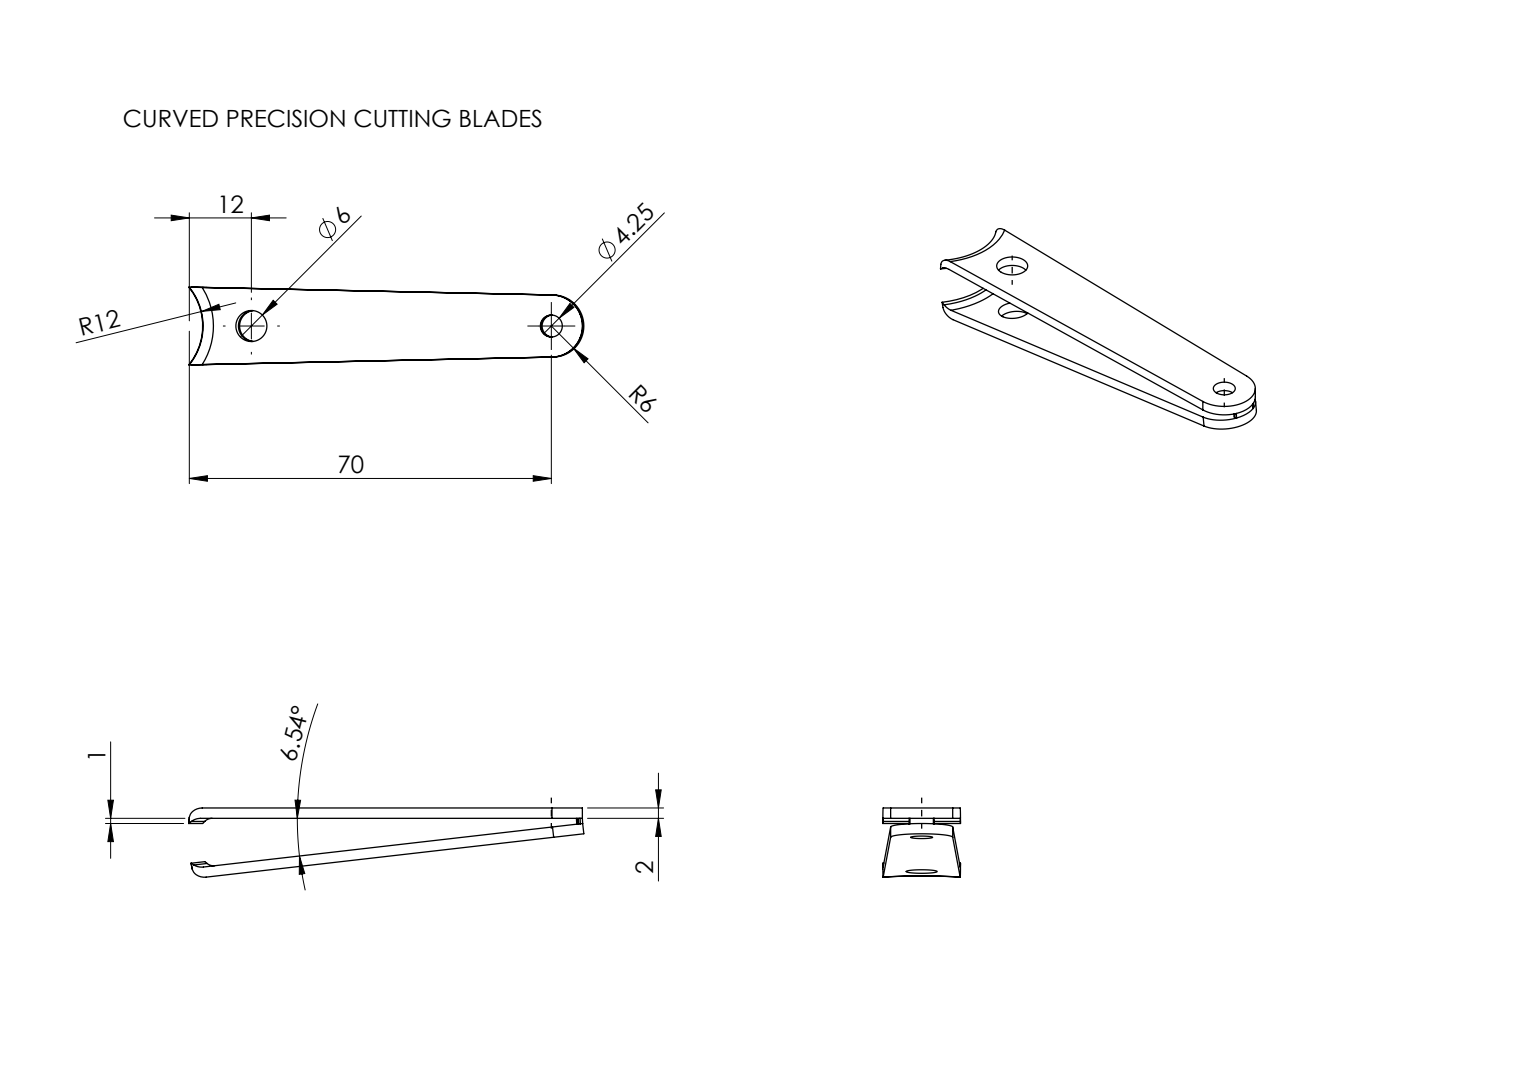
ISO-10303-21;
HEADER;
FILE_DESCRIPTION (('STEP AP214'),
    '1' );
FILE_NAME ('Curved Precision Cutting Blades.step',
    '2026-09-30T04:43:20',
    ( '' ),
    ( '' ),
    'SwSTEP 2.0',
    'SolidWorks 2026',
    '' );
FILE_SCHEMA (( 'AUTOMOTIVE_DESIGN' ));
ENDSEC;

DATA;
#18=VERTEX_POINT ( 'NONE', #46192 ) ;
#27=B_SPLINE_CURVE_WITH_KNOTS ( 'NONE', 3,
 ( #5781, #31047, #23391, #22809, #48941, #35902, #48672, #40707, #18006, #52911, #26803, #36426 ),
 .UNSPECIFIED., .F., .F.,
 ( 4, 2, 2, 2, 2, 4 ),
 ( 0.07980989636644560126, 0.1159099261691615840, 0.2318198523383231402, 0.4636397046766463914, 0.6954595570149695316, 0.9272794093314227215 ),
 .UNSPECIFIED. ) ;
#61=CARTESIAN_POINT ( 'NONE',  ( -69.74692240850775704, 2.000000000000830003, -7.382776467523781250 ) ) ;
#63=ORIENTED_EDGE ( 'NONE', *, *, #47329, .F. ) ;
#89=EDGE_CURVE ( 'NONE', #51823, #2618, #23778, .T. ) ;
#128=ORIENTED_EDGE ( 'NONE', *, *, #52773, .T. ) ;
#145=AXIS2_PLACEMENT_3D ( 'NONE', #38403, #43503, #3755 ) ;
#186=CARTESIAN_POINT ( 'NONE',  ( -66.51694242614880181, -11.33548347488676278, 2.024546322512585039 ) ) ;
#253=ORIENTED_EDGE ( 'NONE', *, *, #19870, .F. ) ;
#280=VERTEX_POINT ( 'NONE', #756 ) ;
#299=DIRECTION ( 'NONE',  ( -0.1139275668495183524, 0.9934890585767659488, 4.694855797473114533E-16 ) ) ;
#354=CARTESIAN_POINT ( 'NONE',  ( -69.95337746243399124, 0.1332479302464926740, -7.442420802399271729 ) ) ;
#433=CARTESIAN_POINT ( 'NONE',  ( 0.4518049228021103203, -3.655895688227122076, 5.998622290806040702 ) ) ;
#492=DIRECTION ( 'NONE',  ( -0.9997703818010067467, 0.000000000000000000, -0.02142857142857158143 ) ) ;
#495=CARTESIAN_POINT ( 'NONE',  ( 4.866417447938704122, 0.000000000000000000, 1.967953638241001002 ) ) ;
#496=CARTESIAN_POINT ( 'NONE',  ( 6.057149706651311583, -1.000000014492634426, -0.7725429650402538817 ) ) ;
#563=VERTEX_POINT ( 'NONE', #20602 ) ;
#641=CARTESIAN_POINT ( 'NONE',  ( -69.63135658628988267, 1.044799017367015193, 7.493821216008851316 ) ) ;
#653=CARTESIAN_POINT ( 'NONE',  ( 4.930947970565944694, -1.129146301979397693, 1.967953638241001446 ) ) ;
#674=ORIENTED_EDGE ( 'NONE', *, *, #1413, .T. ) ;
#685=( BOUNDED_SURFACE ( )  B_SPLINE_SURFACE ( 3, 2, ( 
 ( #15116, #40673, #41213 ),
 ( #40925, #15367, #2009 ),
 ( #44927, #36680, #10586 ),
 ( #28148, #36390, #6041 ),
 ( #45740, #50283, #49989 ),
 ( #19904, #11101, #45457 ),
 ( #10837, #28728, #2308 ),
 ( #24185, #6868, #23354 ),
 ( #1745, #11397, #28423 ),
 ( #45205, #10278, #53441 ),
 ( #19067, #14539, #27899 ),
 ( #6572, #36975, #5739 ),
 ( #23063, #6307, #41503 ),
 ( #54273, #19644, #32439 ),
 ( #32683, #2586, #37220 ),
 ( #53703, #54524, #40385 ),
 ( #49165, #15631, #14818 ),
 ( #32970, #27603, #31853 ),
 ( #1480, #32145, #49470 ),
 ( #18819, #23610, #19344 ),
 ( #53999, #36140, #49740 ),
 ( #23885, #12789, #11933 ),
 ( #42345, #38343, #25300 ),
 ( #33807, #42604, #51427 ),
 ( #41750, #37811, #12527 ),
 ( #7144, #33274, #34109 ),
 ( #3698, #29846, #24716 ),
 ( #54824, #34380, #55668 ) ),
 .UNSPECIFIED., .F., .F., .T. ) 
 B_SPLINE_SURFACE_WITH_KNOTS ( ( 4, 2, 2, 2, 2, 2, 2, 2, 2, 2, 2, 2, 2, 4 ),
 ( 3, 3 ),
 ( 0.005951394764495079696, 0.008223488340404871977, 0.009359535128359769418, 0.01049558191631466512, 0.01276767549222445827, 0.01390372228017935571, 0.01503976906813425142, 0.01617581585608914713, 0.01731186264404404457, 0.01958395621995383598, 0.02072000300790872995, 0.02185604979586362739, 0.02299209658381852484, 0.02412814337177342228 ),
 ( 0.000000000000000000, 1.000000000000000000 ),
 .UNSPECIFIED. ) 
 GEOMETRIC_REPRESENTATION_ITEM ( )  RATIONAL_B_SPLINE_SURFACE ( (
 ( 1.000000000000000000, 0.9218171296615420562, 1.000000000000000000),
 ( 1.000000000000000000, 0.9219582590456437687, 1.000000000000000000),
 ( 1.000000000000000000, 0.9217654209472763149, 1.000000000000000000),
 ( 1.000000000000000000, 0.9218193965238216103, 1.000000000000000000),
 ( 1.000000000000000000, 0.9217886515250015567, 1.000000000000000000),
 ( 1.000000000000000000, 0.9217705453232085677, 1.000000000000000000),
 ( 1.000000000000000000, 0.9217728555239398380, 1.000000000000000000),
 ( 1.000000000000000000, 0.9217839018313299659, 1.000000000000000000),
 ( 1.000000000000000000, 0.9217902773711394993, 1.000000000000000000),
 ( 1.000000000000000000, 0.9218159477363486731, 1.000000000000000000),
 ( 1.000000000000000000, 0.9218381644591753243, 1.000000000000000000),
 ( 1.000000000000000000, 0.9218170478689924341, 1.000000000000000000),
 ( 1.000000000000000000, 0.9218183721981643153, 1.000000000000000000),
 ( 1.000000000000000000, 0.9218243750428467553, 1.000000000000000000),
 ( 1.000000000000000000, 0.9218291361982778875, 1.000000000000000000),
 ( 1.000000000000000000, 0.9218339850783857647, 1.000000000000000000),
 ( 1.000000000000000000, 0.9218340914611712344, 1.000000000000000000),
 ( 1.000000000000000000, 0.9218311426327383540, 1.000000000000000000),
 ( 1.000000000000000000, 0.9218408506515718415, 1.000000000000000000),
 ( 1.000000000000000000, 0.9218298856236216698, 1.000000000000000000),
 ( 1.000000000000000000, 0.9218235216668148047, 1.000000000000000000),
 ( 1.000000000000000000, 0.9218049054835019129, 1.000000000000000000),
 ( 1.000000000000000000, 0.9217926302239767278, 1.000000000000000000),
 ( 1.000000000000000000, 0.9217749384505029564, 1.000000000000000000),
 ( 1.000000000000000000, 0.9217695517188592147, 1.000000000000000000),
 ( 1.000000000000000000, 0.9217886187906866313, 1.000000000000000000),
 ( 1.000000000000000000, 0.9218984684751942993, 1.000000000000000000),
 ( 1.000000000000000000, 0.9217608302862917435, 1.000000000000000000) ) ) 
 REPRESENTATION_ITEM ( '' )  SURFACE ( )  );
#689=CYLINDRICAL_SURFACE ( 'NONE', #24963, 5.241923709989091407 ) ;
#709=CARTESIAN_POINT ( 'NONE',  ( -70.02519189693502710, -0.1222117011752772570, -7.502262482362483276 ) ) ;
#756=CARTESIAN_POINT ( 'NONE',  ( -57.52614991588065152, -8.291364278369169227, 3.000000000000006661 ) ) ;
#761=CARTESIAN_POINT ( 'NONE',  ( -67.73103538350329700, -11.31014138737506336, -7.469194291234003913 ) ) ;
#771=CARTESIAN_POINT ( 'NONE',  ( 6.057149959413268725, -0.9999999855073579136, 0.7725409890818936143 ) ) ;
#933=ADVANCED_FACE ( 'NONE', ( #27544 ), #10224, .F. ) ;
#970=CARTESIAN_POINT ( 'NONE',  ( -69.01437307246155228, -9.005354531669947704, 7.360527835276527320 ) ) ;
#989=ORIENTED_EDGE ( 'NONE', *, *, #52773, .F. ) ;
#994=VERTEX_POINT ( 'NONE', #48574 ) ;
#1008=EDGE_CURVE ( 'NONE', #16356, #25458, #53651, .T. ) ;
#1024=ORIENTED_EDGE ( 'NONE', *, *, #4151, .F. ) ;
#1031=CARTESIAN_POINT ( 'NONE',  ( 5.616557846695583223, -1.037130572669888506, -2.260114876317554700 ) ) ;
#1074=CARTESIAN_POINT ( 'NONE',  ( -66.40205603077350816, -9.309201745752147872, -5.905017180569076096 ) ) ;
#1083=AXIS2_PLACEMENT_3D ( 'NONE', #36884, #36304, #24087 ) ;
#1226=ORIENTED_EDGE ( 'NONE', *, *, #53223, .T. ) ;
#1321=LINE ( 'NONE', #53841, #36634 ) ;
#1336=CARTESIAN_POINT ( 'NONE',  ( -68.94855334729879814, -2.681968279941893282E-15, -7.664179260766972313 ) ) ;
#1352=AXIS2_PLACEMENT_3D ( 'NONE', #55815, #35355, #22001 ) ;
#1364=ORIENTED_EDGE ( 'NONE', *, *, #36334, .T. ) ;
#1379=ORIENTED_EDGE ( 'NONE', *, *, #1008, .F. ) ;
#1413=EDGE_CURVE ( 'NONE', #42953, #21409, #19076, .T. ) ;
#1450=CARTESIAN_POINT ( 'NONE',  ( -67.59744393630020909, -9.446281902138684572, -7.461798308327055373 ) ) ;
#1480=CARTESIAN_POINT ( 'NONE',  ( -67.47740846882294363, -0.6008377845323265021, 3.370402386375713100 ) ) ;
#1529=VERTEX_POINT ( 'NONE', #23332 ) ;
#1540=FILL_AREA_STYLE ('',( #36740 ) ) ;
#1554=CARTESIAN_POINT ( 'NONE',  ( -70.00279782826048347, 0.1332992376639058896, -7.501782499249456393 ) ) ;
#1562=CARTESIAN_POINT ( 'NONE',  ( -67.43178107170270152, -8.821979906182226827, -4.591303796237533597 ) ) ;
#1574=PLANE ( 'NONE',  #11300 ) ;
#1632=CARTESIAN_POINT ( 'NONE',  ( -67.21206727041581530, 2.489116509966271308E-16, 4.722169080041621392 ) ) ;
#1656=DIRECTION ( 'NONE',  ( -0.1139275668495183524, 0.9934890585767659488, 4.694855797473114533E-16 ) ) ;
#1668=B_SPLINE_CURVE_WITH_KNOTS ( 'NONE', 3,
 ( #32011, #15259, #45343, #19212, #36548, #45094, #32574, #44247, #36029, #5608, #5905, #22931, #27771, #6196, #23231, #5351 ),
 .UNSPECIFIED., .F., .F.,
 ( 4, 2, 2, 2, 2, 2, 2, 4 ),
 ( 2.629190268277348252E-18, 0.0004228030555968962517, 0.0008456061111937897929, 0.001268409166790682900, 0.001691212222387575900, 0.002114015277984469116, 0.002536818333581361898, 0.003382424444775107997 ),
 .UNSPECIFIED. ) ;
#1689=CARTESIAN_POINT ( 'NONE',  ( -68.44026216309750055, -1.000000000000000444, 5.059064008999124340 ) ) ;
#1745=CARTESIAN_POINT ( 'NONE',  ( -67.30971128957258998, -0.6012107392119571125, -2.713115426956270060 ) ) ;
#1795=ADVANCED_FACE ( 'NONE', ( #54188 ), #44821, .T. ) ;
#1809=CARTESIAN_POINT ( 'NONE',  ( -66.55839402557589324, -8.722187935008872017, -0.3300946888591901884 ) ) ;
#1857=CARTESIAN_POINT ( 'NONE',  ( 5.221828392167458865, 0.000000000000000000, 2.393421119419573806 ) ) ;
#1904=EDGE_CURVE ( 'NONE', #27821, #18640, #31635, .T. ) ;
#1906=B_SPLINE_CURVE_WITH_KNOTS ( 'NONE', 3,
 ( #20919, #47057, #9009, #51600 ),
 .UNSPECIFIED., .F., .F.,
 ( 4, 4 ),
 ( 0.000000000000000000, 1.000000000000000000 ),
 .UNSPECIFIED. ) ;
#1923=B_SPLINE_CURVE_WITH_KNOTS ( 'NONE', 3,
 ( #45758, #18536, #18837, #36407, #54017, #2023, #19362 ),
 .UNSPECIFIED., .F., .F.,
 ( 4, 3, 4 ),
 ( 0.000000000000000000, 0.0007529153636991639358, 0.001137651663043191038 ),
 .UNSPECIFIED. ) ;
#1979=ORIENTED_EDGE ( 'NONE', *, *, #37264, .T. ) ;
#2003=CARTESIAN_POINT ( 'NONE',  ( -66.84648059262940478, -9.494061817138627291, 1.387855868230217560 ) ) ;
#2009=CARTESIAN_POINT ( 'NONE',  ( -68.06922484120158856, 4.336808689942017736E-15, -7.865887534729849584 ) ) ;
#2018=EDGE_LOOP ( 'NONE', ( #20058, #6656 ) ) ;
#2023=CARTESIAN_POINT ( 'NONE',  ( -69.46128946698341622, -9.665596887234965351, -7.502022462329921204 ) ) ;
#2200=CARTESIAN_POINT ( 'NONE',  ( -68.38969147407715354, -8.931796914766161777, -6.479403174773509910 ) ) ;
#2235=CARTESIAN_POINT ( 'NONE',  ( -69.83802984922479595, -1.000000000000000666, -7.175319846998989171 ) ) ;
#2242=AXIS2_PLACEMENT_3D ( 'NONE', #38054, #38321, #55953 ) ;
#2259=CARTESIAN_POINT ( 'NONE',  ( 5.541166327321979779, -1.059169997729283441, -2.374049323224325825 ) ) ;
#2280=AXIS2_PLACEMENT_3D ( 'NONE', #43032, #43862, #39635 ) ;
#2281=CARTESIAN_POINT ( 'NONE',  ( 5.561339567967533704, -1.056856647418703776, 2.400892578144001366 ) ) ;
#2304=CARTESIAN_POINT ( 'NONE',  ( -67.75769695306428275, -11.47776601246343375, 8.850418579662749252 ) ) ;
#2308=CARTESIAN_POINT ( 'NONE',  ( -66.48098233065147156, 7.155734338404329264E-14, -4.848827299331423646 ) ) ;
#2315=EDGE_CURVE ( 'NONE', #54422, #24558, #36818, .T. ) ;
#2369=CARTESIAN_POINT ( 'NONE',  ( -68.38638472608106156, -9.332867493602380549, 7.478321023991166605 ) ) ;
#2386=CARTESIAN_POINT ( 'NONE',  ( -70.71258200891328727, -0.9999999999999995559, 8.208045577613541255 ) ) ;
#2393=CARTESIAN_POINT ( 'NONE',  ( -68.52794903032595641, 2.000000000000048850, 8.850418579662809648 ) ) ;
#2397=CARTESIAN_POINT ( 'NONE',  ( -69.59783862807636012, -0.6008070088998225255, -7.493102809087827332 ) ) ;
#2446=UNCERTAINTY_MEASURE_WITH_UNIT (LENGTH_MEASURE( 1.000000000000000082E-05 ), #16772, 'distance_accuracy_value', 'NONE');
#2452=CARTESIAN_POINT ( 'NONE',  ( 4.848100717410756211, 0.000000000000000000, -2.029539223447461183 ) ) ;
#2495=CARTESIAN_POINT ( 'NONE',  ( -66.57230477427758331, -8.723772755596309381, -0.6815216469038195557 ) ) ;
#2512=CYLINDRICAL_SURFACE ( 'NONE', #26543, 2.125000000000000000 ) ;
#2541=EDGE_LOOP ( 'NONE', ( #8129, #19924, #8338, #17598 ) ) ;
#2553=CARTESIAN_POINT ( 'NONE',  ( -65.97443392703776510, -1.387778780781445676E-14, 3.266248677641426568 ) ) ;
#2575=CARTESIAN_POINT ( 'NONE',  ( 0.000000000000000000, 0.000000000000000000, -2.125000000000000000 ) ) ;
#2586=CARTESIAN_POINT ( 'NONE',  ( -66.45030873714300412, -4.509921584324644611E-12, 0.7134948435194322647 ) ) ;
#2587=ORIENTED_EDGE ( 'NONE', *, *, #30039, .T. ) ;
#2589=MANIFOLD_SOLID_BREP ( 'Fillet2', #27672 ) ;
#2602=ORIENTED_EDGE ( 'NONE', *, *, #25224, .F. ) ;
#2610=AXIS2_PLACEMENT_3D ( 'NONE', #34638, #13373, #3697 ) ;
#2618=VERTEX_POINT ( 'NONE', #14875 ) ;
#2677=VERTEX_POINT ( 'NONE', #38055 ) ;
#2722=CARTESIAN_POINT ( 'NONE',  ( -68.01236371044051054, -8.487308885305189676, 5.059064008999122564 ) ) ;
#2745=CARTESIAN_POINT ( 'NONE',  ( -67.34291720966972150, -8.812237417047750654, 4.328853820092634308 ) ) ;
#2764=ORIENTED_EDGE ( 'NONE', *, *, #14508, .F. ) ;
#2820=LINE ( 'NONE', #6840, #25906 ) ;
#2876=ORIENTED_EDGE ( 'NONE', *, *, #23935, .F. ) ;
#2901=FACE_OUTER_BOUND ( 'NONE', #30824, .T. ) ;
#2904=CARTESIAN_POINT ( 'NONE',  ( -70.00259797851279586, 0.1329035588801656675, 7.501778215771297553 ) ) ;
#2964=ORIENTED_EDGE ( 'NONE', *, *, #47329, .T. ) ;
#3014=ORIENTED_EDGE ( 'NONE', *, *, #44568, .F. ) ;
#3029=VERTEX_POINT ( 'NONE', #15548 ) ;
#3033=CARTESIAN_POINT ( 'NONE',  ( -67.01351477598909412, -8.774122127324863740, -3.373741216800328235 ) ) ;
#3050=DIRECTION ( 'NONE',  ( -0.9983709377222390602, -0.05705673239519656187, 0.000000000000000000 ) ) ;
#3057=ORIENTED_EDGE ( 'NONE', *, *, #42262, .F. ) ;
#3115=CARTESIAN_POINT ( 'NONE',  ( 5.284365508485809215, -1.088618427183434934, -2.393569053917001810 ) ) ;
#3135=CARTESIAN_POINT ( 'NONE',  ( -68.97404544921916170, -9.738005235595720066, -6.894786738962547901 ) ) ;
#3147=ADVANCED_FACE ( 'NONE', ( #25772 ), #55044, .T. ) ;
#3165=ADVANCED_FACE ( 'NONE', ( #11849, #24934, #38254 ), #42254, .F. ) ;
#3224=EDGE_CURVE ( 'NONE', #21409, #19068, #24895, .T. ) ;
#3229=CARTESIAN_POINT ( 'NONE',  ( -67.91288919400373914, 1.999999999999992673, -8.053057903404074125 ) ) ;
#3234=CARTESIAN_POINT ( 'NONE',  ( -67.13585797164662949, -0.6008874593650106455, 1.683582515887796172 ) ) ;
#3253=DIRECTION ( 'NONE',  ( 0.000000000000000000, 0.000000000000000000, 1.000000000000000000 ) ) ;
#3276=LINE ( 'NONE', #50112, #21456 ) ;
#3295=EDGE_LOOP ( 'NONE', ( #4257, #36445, #3014, #14840 ) ) ;
#3323=CARTESIAN_POINT ( 'NONE',  ( -69.84290760269591658, -9.703778660409923873, -9.299316846403153036 ) ) ;
#3337=CARTESIAN_POINT ( 'NONE',  ( -69.47171822008920117, -0.5008832641493313753, 7.490399608206209869 ) ) ;
#3344=CARTESIAN_POINT ( 'NONE',  ( -66.62858553107250259, -8.730383453837468721, -1.359962337618603412 ) ) ;
#3346=CARTESIAN_POINT ( 'NONE',  ( -69.43561177275644525, -9.791245164465275153, -7.501782499249458169 ) ) ;
#3349=B_SPLINE_CURVE_WITH_KNOTS ( 'NONE', 3,
 ( #54065, #27957, #496, #771, #22637, #34862 ),
 .UNSPECIFIED., .F., .F.,
 ( 4, 2, 4 ),
 ( 0.3753454237082048950, 0.4999999468611081022, 0.6246544700140113093 ),
 .UNSPECIFIED. ) ;
#3353=B_SPLINE_CURVE_WITH_KNOTS ( 'NONE', 3,
 ( #24155, #20137, #37194, #54790, #41474, #2553, #19875, #46543, #55938, #42850, #22116, #30081, #43679, #47692, #30661, #17579, #38895, #26116, #30908, #47961 ),
 .UNSPECIFIED., .F., .F.,
 ( 4, 2, 2, 2, 2, 2, 2, 2, 2, 4 ),
 ( 6.071532165918824830E-18, 0.001980665692890082059, 0.003961331385780158046, 0.005941997078670233599, 0.006932329925115271810, 0.007922662771560309153, 0.009903328464450387308, 0.01188399415734046199, 0.01386465985023053668, 0.01584532554312061484 ),
 .UNSPECIFIED. ) ;
#3361=CARTESIAN_POINT ( 'NONE',  ( -1.246832498358330099E-15, 2.000000000000000000, 0.000000000000000000 ) ) ;
#3365=ORIENTED_EDGE ( 'NONE', *, *, #16323, .F. ) ;
#3443=CARTESIAN_POINT ( 'NONE',  ( -70.00279782826048347, 0.1332992376639058896, -7.501782499249456393 ) ) ;
#3502=( BOUNDED_CURVE ( )  B_SPLINE_CURVE ( 3, ( #14514, #2281, #50256, #36950 ),
 .UNSPECIFIED., .F., .F. ) 
 B_SPLINE_CURVE_WITH_KNOTS ( ( 4, 4 ),
 ( 0.3868401276509516040, 2.001189637452388759 ),
 .UNSPECIFIED. ) 
 CURVE ( )  GEOMETRIC_REPRESENTATION_ITEM ( )  RATIONAL_B_SPLINE_CURVE ( ( 1.000000000000000000, 0.7943613114863611324, 0.7943613114863611324, 1.000000000000000000 ) ) 
 REPRESENTATION_ITEM ( '' )  );
#3508=DIRECTION ( 'NONE',  ( 0.000000000000000000, 0.000000000000000000, -1.000000000000000000 ) ) ;
#3512=CARTESIAN_POINT ( 'NONE',  ( -68.03033152755355673, 2.000000000000001332, -8.215550190268007924 ) ) ;
#3515=CARTESIAN_POINT ( 'NONE',  ( -68.33274616240578325, -0.6011730142051754378, 5.504334939579325514 ) ) ;
#3559=ADVANCED_BREP_SHAPE_REPRESENTATION ( '', ( #2589, #2610 ), #47980 ) ;
#3586=CARTESIAN_POINT ( 'NONE',  ( -68.40341787366602944, -9.538706321749058858, -7.664179260766974089 ) ) ;
#3590=ORIENTED_EDGE ( 'NONE', *, *, #23040, .F. ) ;
#3596=ORIENTED_EDGE ( 'NONE', *, *, #45911, .T. ) ;
#3597=ORIENTED_EDGE ( 'NONE', *, *, #44568, .T. ) ;
#3603=CARTESIAN_POINT ( 'NONE',  ( -69.59775774058348929, -0.6007421665236040154, 7.493101075386322307 ) ) ;
#3625=DIRECTION ( 'NONE',  ( -0.05705673239519650636, 0.9983709377222390602, 2.351258244848514932E-16 ) ) ;
#3627=CARTESIAN_POINT ( 'NONE',  ( -70.19153117219258320, -11.75686401390256464, -8.809708619959531362 ) ) ;
#3637=PRODUCT_CONTEXT ( 'NONE', #12626, 'mechanical' ) ;
#3658=VERTEX_POINT ( 'NONE', #26832 ) ;
#3662=CARTESIAN_POINT ( 'NONE',  ( -65.13109422105631552, -9.163455212069004929, 1.319813854473150805 ) ) ;
#3697=DIRECTION ( 'NONE',  ( 1.000000000000000000, 0.000000000000000000, 0.000000000000000000 ) ) ;
#3698=CARTESIAN_POINT ( 'NONE',  ( -69.44698877097060574, -0.5991245381873403497, 7.306242118358709625 ) ) ;
#3755=DIRECTION ( 'NONE',  ( -2.710505431213760161E-17, 4.336808689942016257E-16, -1.000000000000000000 ) ) ;
#3775=CARTESIAN_POINT ( 'NONE',  ( -68.15687750496505259, 0.1329650153340585228, 4.357869429823836960 ) ) ;
#3778=CARTESIAN_POINT ( 'NONE',  ( -67.13280394075316337, -0.6010134810807099548, -1.671631898859742060 ) ) ;
#3779=CARTESIAN_POINT ( 'NONE',  ( 5.618093942130458096, -1.050357310661657939, 2.260478214906367800 ) ) ;
#3839=CARTESIAN_POINT ( 'NONE',  ( 2.602374448188125350E-16, 2.000000000000000000, 2.125000000000000000 ) ) ;
#3853=VECTOR ( 'NONE', #15237, 1000.000000000000114 ) ;
#4013=ORIENTED_EDGE ( 'NONE', *, *, #29746, .F. ) ;
#4051=ADVANCED_FACE ( 'NONE', ( #15363 ), #15130, .T. ) ;
#4053=CARTESIAN_POINT ( 'NONE',  ( -68.61315424319464285, 1.787077962669009867, 7.471997583267850018 ) ) ;
#4073=CARTESIAN_POINT ( 'NONE',  ( -69.63118656663708350, 0.1323540994886103217, 7.053755868282808983 ) ) ;
#4078=CARTESIAN_POINT ( 'NONE',  ( -67.30049973920597495, -0.6012074100331669113, -2.670129092015942618 ) ) ;
#4087=CARTESIAN_POINT ( 'NONE',  ( -70.10169143752739274, -0.9999999999999995559, 7.503902134509972122 ) ) ;
#4091=AXIS2_PLACEMENT_3D ( 'NONE', #42033, #28725, #25023 ) ;
#4130=CARTESIAN_POINT ( 'NONE',  ( 5.058454994527578741, -1.127275664452432880, 2.289010529401726224 ) ) ;
#4151=EDGE_CURVE ( 'NONE', #994, #45407, #14068, .T. ) ;
#4167=VECTOR ( 'NONE', #11631, 1000.000000000000000 ) ;
#4217=EDGE_LOOP ( 'NONE', ( #48865, #43698, #34137, #17569 ) ) ;
#4219=VERTEX_POINT ( 'NONE', #34636 ) ;
#4246=CARTESIAN_POINT ( 'NONE',  ( -66.78407322188951412, -9.486793844097082484, -0.6948190221874483985 ) ) ;
#4257=ORIENTED_EDGE ( 'NONE', *, *, #55337, .F. ) ;
#4274=EDGE_CURVE ( 'NONE', #16523, #563, #8992, .T. ) ;
#4368=FACE_OUTER_BOUND ( 'NONE', #16584, .T. ) ;
#4371=CARTESIAN_POINT ( 'NONE',  ( -67.21057658696469161, 2.000000000012947865, 0.7018102913198165371 ) ) ;
#4404=ORIENTED_EDGE ( 'NONE', *, *, #89, .F. ) ;
#4407=B_SPLINE_CURVE_WITH_KNOTS ( 'NONE', 3,
 ( #45023, #27980, #32239, #53517, #40486, #10672 ),
 .UNSPECIFIED., .F., .F.,
 ( 4, 2, 4 ),
 ( 0.05059699584195882782, 0.5000000368888000146, 0.9494030779356412708 ),
 .UNSPECIFIED. ) ;
#4455=B_SPLINE_CURVE_WITH_KNOTS ( 'NONE', 3,
 ( #43486, #1450, #40349, #5432, #35821, #4867 ),
 .UNSPECIFIED., .F., .F.,
 ( 4, 2, 4 ),
 ( 1.387778780781430114E-17, 0.0009531277170912127008, 0.001906255434182411524 ),
 .UNSPECIFIED. ) ;
#4476=ADVANCED_FACE ( 'NONE', ( #48370 ), #9480, .T. ) ;
#4483=CARTESIAN_POINT ( 'NONE',  ( -68.45530293218364193, -11.55776342273651380, -6.702751532743291385 ) ) ;
#4484=ORIENTED_EDGE ( 'NONE', *, *, #1904, .T. ) ;
#4506=CARTESIAN_POINT ( 'NONE',  ( -67.70222436837769919, -9.592143523249529125, 4.605078063924984200 ) ) ;
#4511=EDGE_CURVE ( 'NONE', #5292, #43677, #38586, .T. ) ;
#4538=VERTEX_POINT ( 'NONE', #6614 ) ;
#4617=CARTESIAN_POINT ( 'NONE',  ( 4.918891891700034158, -1.130528823225185109, 1.997863978257570228 ) ) ;
#4653=( BOUNDED_SURFACE ( )  B_SPLINE_SURFACE ( 3, 2, ( 
 ( #2393, #19719, #37043 ),
 ( #54345, #51208, #4073 ),
 ( #16279, #33600, #34724 ),
 ( #25113, #25373, #34195 ),
 ( #38733, #8620, #51507 ),
 ( #42674, #29917, #52041 ),
 ( #17397, #13156, #3775 ),
 ( #8323, #21405, #20562 ),
 ( #25641, #21096, #38424 ),
 ( #43280, #42969, #47216 ),
 ( #12600, #4371, #55750 ),
 ( #56045, #30494, #17138 ),
 ( #25951, #21681, #46662 ),
 ( #7786, #7479, #51758 ),
 ( #46962, #12012, #55189 ),
 ( #42421, #50910, #29663 ),
 ( #38995, #16864, #47508 ),
 ( #37885, #34448, #24803 ),
 ( #29350, #42123, #30190 ),
 ( #3229, #12868, #12323 ),
 ( #3512, #8063, #20821 ),
 ( #38139, #61, #55457 ),
 ( #16556, #33892, #354 ),
 ( #18828, #22234, #9161 ) ),
 .UNSPECIFIED., .F., .F., .F. ) 
 B_SPLINE_SURFACE_WITH_KNOTS ( ( 4, 2, 2, 2, 2, 2, 2, 2, 2, 2, 2, 4 ),
 ( 3, 3 ),
 ( 0.008994972463978564287, 0.01138926720843922921, 0.01258641458066956167, 0.01378356195289989587, 0.01617785669736056253, 0.01857215144182122746, 0.02096644618628189238, 0.02336074093074255731, 0.02575503567520322223, 0.02695218304743355470, 0.02755075673354872093, 0.02814933041966388716 ),
 ( 0.000000000000000000, 1.000000000000000000 ),
 .UNSPECIFIED. ) 
 GEOMETRIC_REPRESENTATION_ITEM ( )  RATIONAL_B_SPLINE_SURFACE ( (
 ( 1.000000000000000000, 0.7302382283600404866, 1.000000000000000000),
 ( 1.000000000000000000, 0.7302057701444414350, 1.000000000000000000),
 ( 1.000000000000000000, 0.7302261543189000337, 1.000000000000000000),
 ( 1.000000000000000000, 0.7302340627759330571, 1.000000000000000000),
 ( 1.000000000000000000, 0.7302358193534487230, 1.000000000000000000),
 ( 1.000000000000000000, 0.7302356584982084842, 1.000000000000000000),
 ( 1.000000000000000000, 0.7302336981036621211, 1.000000000000000000),
 ( 1.000000000000000000, 0.7302244465159644093, 1.000000000000000000),
 ( 1.000000000000000000, 0.7302382397051314644, 1.000000000000000000),
 ( 1.000000000000000000, 0.7302438375851851848, 1.000000000000000000),
 ( 1.000000000000000000, 0.7302379409314863068, 1.000000000000000000),
 ( 1.000000000000000000, 0.7302249128351889773, 1.000000000000000000),
 ( 1.000000000000000000, 0.7302266904876862919, 1.000000000000000000),
 ( 1.000000000000000000, 0.7302305284562681242, 1.000000000000000000),
 ( 1.000000000000000000, 0.7302278475313366268, 1.000000000000000000),
 ( 1.000000000000000000, 0.7302208473858853299, 1.000000000000000000),
 ( 1.000000000000000000, 0.7302205818823860328, 1.000000000000000000),
 ( 1.000000000000000000, 0.7302413824363716000, 1.000000000000000000),
 ( 1.000000000000000000, 0.7302489349993748213, 1.000000000000000000),
 ( 1.000000000000000000, 0.7302381596253557650, 1.000000000000000000),
 ( 1.000000000000000000, 0.7302138215221798401, 1.000000000000000000),
 ( 1.000000000000000000, 0.7302588551337141354, 1.000000000000000000),
 ( 1.000000000000000000, 0.7302821861416568527, 1.000000000000000000),
 ( 1.000000000000000000, 0.7303030204721981944, 1.000000000000000000) ) ) 
 REPRESENTATION_ITEM ( '' )  SURFACE ( )  );
#4694=ORIENTED_EDGE ( 'NONE', *, *, #37182, .T. ) ;
#4735=CARTESIAN_POINT ( 'NONE',  ( -66.74342152241241877, -11.36145478494482042, -7.448289400635804469 ) ) ;
#4751=CARTESIAN_POINT ( 'NONE',  ( 0.1285714285714296967, 2.000000000000000000, 5.998622290806041590 ) ) ;
#4867=CARTESIAN_POINT ( 'NONE',  ( -69.11692417668358246, -9.015782624321049710, -7.493102809087829108 ) ) ;
#4900=FACE_OUTER_BOUND ( 'NONE', #19248, .T. ) ;
#4917=CARTESIAN_POINT ( 'NONE',  ( 0.2239497891030729493, -1.668917571073590622, 5.998622290806042479 ) ) ;
#4942=ORIENTED_EDGE ( 'NONE', *, *, #45650, .F. ) ;
#5034=CARTESIAN_POINT ( 'NONE',  ( -67.31362796205407051, -11.38444644600729738, -7.460487485314824418 ) ) ;
#5038=CIRCLE ( 'NONE', #36775, 3.000000000000001332 ) ;
#5088=ORIENTED_EDGE ( 'NONE', *, *, #24847, .F. ) ;
#5094=ORIENTED_EDGE ( 'NONE', *, *, #23221, .F. ) ;
#5139=DIRECTION ( 'NONE',  ( 0.9932609354084158682, 0.1139014070068027351, -0.02142857142857155367 ) ) ;
#5216=CARTESIAN_POINT ( 'NONE',  ( -66.84137242167658144, 1.999999999999978018, 6.312544413184001613 ) ) ;
#5225=CARTESIAN_POINT ( 'NONE',  ( 4.848100717410752658, 0.000000000000000000, 2.061810099490657411 ) ) ;
#5242=DIRECTION ( 'NONE',  ( -0.9983709377222389492, -0.05705673239519657575, 0.000000000000000000 ) ) ;
#5271=CARTESIAN_POINT ( 'NONE',  ( -66.83595559056652746, -8.754112661980432364, 2.678990660366957322 ) ) ;
#5292=VERTEX_POINT ( 'NONE', #22183 ) ;
#5351=CARTESIAN_POINT ( 'NONE',  ( -67.50702643244157741, 2.000000000000000000, -7.448289400635801805 ) ) ;
#5373=FACE_OUTER_BOUND ( 'NONE', #42581, .T. ) ;
#5413=DIRECTION ( 'NONE',  ( 0.9997703818010067467, 0.000000000000000000, 0.02142857142857158143 ) ) ;
#5432=CARTESIAN_POINT ( 'NONE',  ( -68.54375487892276908, -9.299823415457391107, -7.481591365497658686 ) ) ;
#5453=CARTESIAN_POINT ( 'NONE',  ( -64.66143966744172644, -11.12270517324659735, 1.620203490756831677 ) ) ;
#5465=EDGE_CURVE ( 'NONE', #9189, #4538, #41921, .T. ) ;
#5477=ORIENTED_EDGE ( 'NONE', *, *, #55930, .F. ) ;
#5486=ORIENTED_EDGE ( 'NONE', *, *, #30197, .T. ) ;
#5509=PRESENTATION_STYLE_ASSIGNMENT (( #48956 ) ) ;
#5601=CARTESIAN_POINT ( 'NONE',  ( -69.18604761972393646, -0.9999999999995238253, 6.394134653913046584 ) ) ;
#5608=CARTESIAN_POINT ( 'NONE',  ( -68.99560423633737116, 1.595632167476292107, -7.480194822499073304 ) ) ;
#5671=CARTESIAN_POINT ( 'NONE',  ( 0.4518049228021103203, -3.655895688227122076, 5.998622290806040702 ) ) ;
#5684=EDGE_LOOP ( 'NONE', ( #19261, #32006, #1364, #35597 ) ) ;
#5734=CARTESIAN_POINT ( 'NONE',  ( -65.67591093208449138, -11.23903885787223267, -5.460169066039067154 ) ) ;
#5739=CARTESIAN_POINT ( 'NONE',  ( -65.60880995838058993, 5.724587470723463412E-14, -0.7600040867678790057 ) ) ;
#5781=CARTESIAN_POINT ( 'NONE',  ( -69.66347483736342383, -8.676648739292067702, -7.503912900124009688 ) ) ;
#5813=CARTESIAN_POINT ( 'NONE',  ( -70.01399353402076997, 0.005543651780989746099, -7.502022462329923869 ) ) ;
#5856=AXIS2_PLACEMENT_3D ( 'NONE', #20019, #29708, #29399 ) ;
#5873=CARTESIAN_POINT ( 'NONE',  ( 5.057731014323088026, -1.114607557371864122, 2.289010529401726668 ) ) ;
#5884=CARTESIAN_POINT ( 'NONE',  ( -69.89574092751220746, 0.1327608315404790740, 7.370754069753728821 ) ) ;
#5899=CARTESIAN_POINT ( 'NONE',  ( -70.39747693292142117, -1.183819181302419339E-15, -9.299316846403151260 ) ) ;
#5905=CARTESIAN_POINT ( 'NONE',  ( -68.87092941434458737, 1.666157950113242636, -7.477522605581019555 ) ) ;
#5936=CARTESIAN_POINT ( 'NONE',  ( 0.3240706152708106025, -3.670543518250628967, -1.335466778558061241E-15 ) ) ;
#6037=CARTESIAN_POINT ( 'NONE',  ( -68.68358996202969990, -9.704760845431907867, -6.471852447744065095 ) ) ;
#6041=CARTESIAN_POINT ( 'NONE',  ( -67.10382889302627518, 2.688821387764050996E-14, -6.245432549308967296 ) ) ;
#6112=VECTOR ( 'NONE', #41220, 1000.000000000000000 ) ;
#6121=CARTESIAN_POINT ( 'NONE',  ( -67.86011035204582242, -8.871290095601276349, 5.504334939579316632 ) ) ;
#6156=EDGE_CURVE ( 'NONE', #11345, #18640, #27, .T. ) ;
#6196=CARTESIAN_POINT ( 'NONE',  ( -68.07613967535824884, 1.957879731433807224, -7.460487485314824418 ) ) ;
#6217=CARTESIAN_POINT ( 'NONE',  ( -68.75873835633035469, -8.975997488099570987, -7.041125024101304142 ) ) ;
#6235=EDGE_LOOP ( 'NONE', ( #12749, #11486, #2764, #49889, #8798, #34469, #63 ) ) ;
#6250=CARTESIAN_POINT ( 'NONE',  ( -69.30403031588791407, -1.000000000000000666, -6.450409451741321298 ) ) ;
#6283=CARTESIAN_POINT ( 'NONE',  ( 4.866417447938705898, 0.000000000000000000, -1.967953638240998337 ) ) ;
#6284=COLOUR_RGB ( '', 0.66274510, 0.83137255, 0.94901961) ;
#6303=CARTESIAN_POINT ( 'NONE',  ( -66.80596856838349140, -11.36862731764621515, 7.586268967159024434 ) ) ;
#6307=CARTESIAN_POINT ( 'NONE',  ( -66.43438701333805341, -1.405445106517288831E-11, -0.3573205173190009409 ) ) ;
#6348=ORIENTED_EDGE ( 'NONE', *, *, #49291, .T. ) ;
#6390=CARTESIAN_POINT ( 'NONE',  ( -1.246832498358330099E-15, 0.000000000000000000, 0.000000000000000000 ) ) ;
#6392=CARTESIAN_POINT ( 'NONE',  ( 5.415767943939227891, -1.059274754233117344, -2.423176835373680227 ) ) ;
#6451=CARTESIAN_POINT ( 'NONE',  ( 5.057731014323088026, -1.114607557371864122, 2.289010529401726668 ) ) ;
#6475=CARTESIAN_POINT ( 'NONE',  ( -67.11552282731028640, -9.391017982635339933, -7.239294561908663717 ) ) ;
#6567=CARTESIAN_POINT ( 'NONE',  ( -66.91943787661757881, -11.38163932023507385, -3.410887992466311136 ) ) ;
#6572=CARTESIAN_POINT ( 'NONE',  ( -67.03651911971512334, -0.6010133214110180422, -0.6815216469086778917 ) ) ;
#6614=CARTESIAN_POINT ( 'NONE',  ( 4.994031378522667985, 0.000000000000000000, 2.289010529401726668 ) ) ;
#6648=CARTESIAN_POINT ( 'NONE',  ( -67.56320601492518563, -0.9999999999999974465, -2.442027903730110250 ) ) ;
#6652=FACE_OUTER_BOUND ( 'NONE', #24701, .T. ) ;
#6656=ORIENTED_EDGE ( 'NONE', *, *, #9049, .T. ) ;
#6670=CARTESIAN_POINT ( 'NONE',  ( -69.43545830293986398, -9.790829293527439248, 7.501778215771295777 ) ) ;
#6675=ORIENTED_EDGE ( 'NONE', *, *, #52380, .T. ) ;
#6759=CARTESIAN_POINT ( 'NONE',  ( -65.07086784306864047, -9.156548800121029785, 0.3806443636437001898 ) ) ;
#6806=VECTOR ( 'NONE', #5139, 1000.000000000000114 ) ;
#6816=ADVANCED_FACE ( 'NONE', ( #5373 ), #39453, .T. ) ;
#6840=CARTESIAN_POINT ( 'NONE',  ( 0.1285714285714296967, 2.000000000000000000, 5.998622290806041590 ) ) ;
#6864=CARTESIAN_POINT ( 'NONE',  ( -69.49918034145071033, -9.798606072444741244, -7.579899494734580578 ) ) ;
#6868=CARTESIAN_POINT ( 'NONE',  ( -66.91434672699239172, 8.085008987418439830E-12, -3.536654368688153305 ) ) ;
#6927=ORIENTED_EDGE ( 'NONE', *, *, #36562, .T. ) ;
#6945=CARTESIAN_POINT ( 'NONE',  ( -67.84970284451081568, 2.000000000000001776, -4.138470222184130520 ) ) ;
#7023=DIRECTION ( 'NONE',  ( 0.000000000000000000, -5.782411586589354681E-16, 1.000000000000000000 ) ) ;
#7052=CARTESIAN_POINT ( 'NONE',  ( -65.97914594675513911, -9.260704868562440240, -1.425848428488597053 ) ) ;
#7084=VERTEX_POINT ( 'NONE', #21519 ) ;
#7111=CARTESIAN_POINT ( 'NONE',  ( -66.91760232564914190, -9.368321606677067592, -6.901381173728423413 ) ) ;
#7129=ORIENTED_EDGE ( 'NONE', *, *, #44539, .F. ) ;
#7140=CARTESIAN_POINT ( 'NONE',  ( -67.75725311154501185, -11.47771511529060007, -8.849861037685116116 ) ) ;
#7144=CARTESIAN_POINT ( 'NONE',  ( -69.24996902294029155, -0.6012229694362068999, 7.030741166005281428 ) ) ;
#7292=CARTESIAN_POINT ( 'NONE',  ( -67.81626209598535127, 0.000000000000000000, 7.454917401049828918 ) ) ;
#7302=CARTESIAN_POINT ( 'NONE',  ( -68.96686481439014926, -9.000268183362885921, 7.306242118345172898 ) ) ;
#7474=CARTESIAN_POINT ( 'NONE',  ( -67.98273966911209243, -0.9999999999999978906, -3.909888324369924284 ) ) ;
#7479=CARTESIAN_POINT ( 'NONE',  ( -67.50629308046563892, 1.999999999992078781, -2.738438791729908228 ) ) ;
#7563=CARTESIAN_POINT ( 'NONE',  ( -68.57937869370883277, -9.558884488700273963, 7.875383342262417763 ) ) ;
#7586=CARTESIAN_POINT ( 'NONE',  ( -65.31549755956690717, -11.19770874131334182, 4.495433075559887470 ) ) ;
#7589=CARTESIAN_POINT ( 'NONE',  ( -65.92002855750158119, -9.253925629004317699, -0.7138195548257249001 ) ) ;
#7602=DIRECTION ( 'NONE',  ( -0.05705673239519651330, 0.9983709377222391712, 2.351258244848514932E-16 ) ) ;
#7635=DIRECTION ( 'NONE',  ( -0.1139275668495183386, 0.9934890585767658377, 4.694855797473113547E-16 ) ) ;
#7651=ORIENTED_EDGE ( 'NONE', *, *, #13029, .T. ) ;
#7654=CARTESIAN_POINT ( 'NONE',  ( -66.04895207021591830, -9.268709830190596577, 5.126821739293232483 ) ) ;
#7735=AXIS2_PLACEMENT_3D ( 'NONE', #11713, #33315, #15406 ) ;
#7753=CARTESIAN_POINT ( 'NONE',  ( -57.29829478218162109, -10.27834239552269757, 4.211285351864063224E-15 ) ) ;
#7786=CARTESIAN_POINT ( 'NONE',  ( -65.68175713575769237, 2.000000000000022204, -3.167379070712565969 ) ) ;
#7825=VERTEX_POINT ( 'NONE', #51664 ) ;
#7841=FACE_OUTER_BOUND ( 'NONE', #31554, .T. ) ;
#7902=CARTESIAN_POINT ( 'NONE',  ( -66.72811894189939608, -9.346592750493281088, 4.538413701023873870 ) ) ;
#8063=CARTESIAN_POINT ( 'NONE',  ( -69.53894961980590494, 1.999999999999173550, -7.108028418033228490 ) ) ;
#8071=AXIS2_PLACEMENT_3D ( 'NONE', #38134, #42964, #3508 ) ;
#8129=ORIENTED_EDGE ( 'NONE', *, *, #47519, .T. ) ;
#8133=DIRECTION ( 'NONE',  ( -2.710505431213760161E-17, 4.336808689942016257E-16, -1.000000000000000000 ) ) ;
#8138=CARTESIAN_POINT ( 'NONE',  ( -68.75329340164451253, -8.572274407770867910, 6.394134653913044808 ) ) ;
#8178=CARTESIAN_POINT ( 'NONE',  ( -70.57153585115312922, -8.780779913117141788, -8.550077602493740159 ) ) ;
#8183=FACE_OUTER_BOUND ( 'NONE', #22695, .T. ) ;
#8197=CARTESIAN_POINT ( 'NONE',  ( 4.912750499197526821, -1.131233082521083455, -2.061810099490656079 ) ) ;
#8212=DIRECTION ( 'NONE',  ( -0.000000000000000000, -1.000000000000000000, -0.000000000000000000 ) ) ;
#8323=CARTESIAN_POINT ( 'NONE',  ( -65.89105554006435739, 1.999999999999976685, 3.962576710808226377 ) ) ;
#8326=CARTESIAN_POINT ( 'NONE',  ( -67.91322597425605068, -0.6009552942202146530, 4.584835828370202648 ) ) ;
#8338=ORIENTED_EDGE ( 'NONE', *, *, #15832, .T. ) ;
#8422=CARTESIAN_POINT ( 'NONE',  ( 4.848100717410755323, 0.000000000000000000, -2.162384853247615535 ) ) ;
#8448=CARTESIAN_POINT ( 'NONE',  ( -70.12381838982661009, -8.729438269679169693, -8.047023921085742160 ) ) ;
#8562=VECTOR ( 'NONE', #56184, 1000.000000000000114 ) ;
#8620=CARTESIAN_POINT ( 'NONE',  ( -68.46813845749102256, 2.000000000003206324, 5.359670781636787673 ) ) ;
#8624=VECTOR ( 'NONE', #24911, 1000.000000000000114 ) ;
#8649=AXIS2_PLACEMENT_3D ( 'NONE', #17485, #12103, #33980 ) ;
#8711=DIRECTION ( 'NONE',  ( -0.1139275668495183386, 0.9934890585767658377, 4.694855797473113547E-16 ) ) ;
#8758=CARTESIAN_POINT ( 'NONE',  ( 0.3726814890124213187, -6.521129970779321994, -1.535787955176781389E-15 ) ) ;
#8761=CARTESIAN_POINT ( 'NONE',  ( -67.08542992444135677, -8.381013491352103273, 2.158836163547856124 ) ) ;
#8798=ORIENTED_EDGE ( 'NONE', *, *, #15832, .F. ) ;
#8809=EDGE_CURVE ( 'NONE', #53459, #16329, #30715, .T. ) ;
#8840=( NAMED_UNIT ( * ) PLANE_ANGLE_UNIT ( ) SI_UNIT ( $, .RADIAN. ) );
#8945=VERTEX_POINT ( 'NONE', #44930 ) ;
#8992=B_SPLINE_CURVE_WITH_KNOTS ( 'NONE', 3,
 ( #20664, #12696, #42239, #37704, #42518, #41655, #16970, #55027, #37391, #11582, #16118, #7586, #29458, #51325, #55561, #24914 ),
 .UNSPECIFIED., .F., .F.,
 ( 4, 2, 2, 2, 2, 2, 2, 4 ),
 ( 3.469446951953618041E-18, 0.001965516910292332883, 0.003931033820584662296, 0.007862067641169319387, 0.009827584551461647500, 0.01179310146175397735, 0.01375861837204630372, 0.01572413528233863184 ),
 .UNSPECIFIED. ) ;
#8994=ORIENTED_EDGE ( 'NONE', *, *, #45650, .T. ) ;
#9009=CARTESIAN_POINT ( 'NONE',  ( 5.488878160879001378, 0.000000000000000000, 2.420140035803472589 ) ) ;
#9023=CARTESIAN_POINT ( 'NONE',  ( -68.15152480690021264, -11.52292790806604117, 6.355103916287435872 ) ) ;
#9049=EDGE_CURVE ( 'NONE', #18417, #12427, #47187, .T. ) ;
#9055=ADVANCED_FACE ( 'NONE', ( #47429 ), #50584, .T. ) ;
#9161=CARTESIAN_POINT ( 'NONE',  ( -70.06679111606356969, 0.1333700068432634167, -7.579899494734611665 ) ) ;
#9181=CARTESIAN_POINT ( 'NONE',  ( -69.29909153375579933, -8.902711886016962950, -7.496705766434924811 ) ) ;
#9189=VERTEX_POINT ( 'NONE', #21612 ) ;
#9195=CARTESIAN_POINT ( 'NONE',  ( 0.3726814890124213187, -6.521129970779321994, -1.535787955176781389E-15 ) ) ;
#9237=DIRECTION ( 'NONE',  ( -0.05705673239519651330, 0.9983709377222391712, 2.351258244848514932E-16 ) ) ;
#9238=CARTESIAN_POINT ( 'NONE',  ( 5.585384064119276459, -1.054099363964956737, -2.341019274736492850 ) ) ;
#9239=EDGE_CURVE ( 'NONE', #17419, #22456, #13957, .T. ) ;
#9284=CARTESIAN_POINT ( 'NONE',  ( 5.618587682346595003, -1.056427131421802557, -2.260561881690064556 ) ) ;
#9289=DIRECTION ( 'NONE',  ( -0.000000000000000000, -1.000000000000000000, -0.000000000000000000 ) ) ;
#9292=COLOUR_RGB ( '', 0.66274510, 0.83137255, 0.94901961) ;
#9306=EDGE_CURVE ( 'NONE', #45407, #994, #51771, .T. ) ;
#9329=ORIENTED_EDGE ( 'NONE', *, *, #24412, .T. ) ;
#9335=ORIENTED_EDGE ( 'NONE', *, *, #41113, .T. ) ;
#9453=CARTESIAN_POINT ( 'NONE',  ( -65.52441736963763219, 2.000000000000033751, -2.612833193080994043 ) ) ;
#9480=PLANE ( 'NONE',  #34990 ) ;
#9575=CARTESIAN_POINT ( 'NONE',  ( 4.912750499197525045, -1.131233082521085898, 2.162384853247616867 ) ) ;
#9592=CARTESIAN_POINT ( 'NONE',  ( 5.518152842597062069, -1.042152011631011899, -2.501942471198983942 ) ) ;
#9637=CARTESIAN_POINT ( 'NONE',  ( -68.21250092108449792, -9.516813072189039602, -7.380886937840050344 ) ) ;
#9888=B_SPLINE_CURVE_WITH_KNOTS ( 'NONE', 3,
 ( #25356, #42658, #21076, #42947, #4053, #27039, #30745, #23344, #35285, #22507, #641, #18808, #27591, #17962 ),
 .UNSPECIFIED., .F., .F.,
 ( 4, 2, 2, 2, 2, 2, 4 ),
 ( 1.404617285391336434E-17, 0.0008437472854879493047, 0.001265620928231936696, 0.001687494570975924197, 0.002109368213719911046, 0.002531241856463898980, 0.003374989141951896966 ),
 .UNSPECIFIED. ) ;
#9894=CARTESIAN_POINT ( 'NONE',  ( -67.06923785704015017, -9.519576449723603062, 2.681528892132509334 ) ) ;
#9948=CARTESIAN_POINT ( 'NONE',  ( 4.918891891700036822, -1.130528823225183332, -1.997863978257569118 ) ) ;
#9994=CARTESIAN_POINT ( 'NONE',  ( -69.18949689463744335, -11.64195653086973614, 7.657023247222856099 ) ) ;
#10022=CARTESIAN_POINT ( 'NONE',  ( 4.848100717410752658, 0.000000000000000000, 2.162384853247617311 ) ) ;
#10113=EDGE_LOOP ( 'NONE', ( #33204, #8994, #23226, #34217, #10623, #49393, #45235 ) ) ;
#10125=CARTESIAN_POINT ( 'NONE',  ( -69.14205738506272780, 0.1323226647188939231, -6.443496511055998965 ) ) ;
#10131=B_SPLINE_SURFACE_WITH_KNOTS ( 'NONE', 1, 3, ( 
 ( #3627, #21792, #47342, #4483, #29775, #33718, #34564, #26326, #186, #42536, #9023, #43387, #43639, #20683 ),
 ( #8178, #8448, #37998, #42794, #38257, #34865, #25776, #38848, #8761, #17243, #25486, #51880, #55581, #29480 ) ),
 .UNSPECIFIED., .F., .F., .F.,
 ( 2, 2 ),
 ( 4, 2, 2, 2, 2, 2, 4 ),
 ( 0.000000000000000000, 1.000000000000000000 ),
 ( 0.000000000000000000, 0.1159099261691615840, 0.2318198523383231680, 0.4636397046766463359, 0.6954595570149695316, 0.9272794093532926718, 1.000000000000000000 ),
 .UNSPECIFIED. ) ;
#10163=EDGE_LOOP ( 'NONE', ( #25777, #34390, #38768, #26916 ) ) ;
#10192=EDGE_CURVE ( 'NONE', #13134, #33706, #54610, .T. ) ;
#10202=CARTESIAN_POINT ( 'NONE',  ( 5.204999356530675136, -6.244963811491316186, -2.061810099490657411 ) ) ;
#10224=PLANE ( 'NONE',  #33184 ) ;
#10274=CARTESIAN_POINT ( 'NONE',  ( -68.50280060959401851, -9.683984559439076989, -6.182688104189539402 ) ) ;
#10278=CARTESIAN_POINT ( 'NONE',  ( -66.55406810601930090, 5.346159682976206314E-12, -1.783245832580018675 ) ) ;
#10293=CARTESIAN_POINT ( 'NONE',  ( -66.84075661360076026, 2.000000000000022204, -6.315096454939387094 ) ) ;
#10358=CARTESIAN_POINT ( 'NONE',  ( -66.57353123603060396, -8.724002626923901715, 0.6758588499069799749 ) ) ;
#10380=VERTEX_POINT ( 'NONE', #39576 ) ;
#10477=CARTESIAN_POINT ( 'NONE',  ( -66.09197391315379377, -9.273643325778634150, -5.205015551674848417 ) ) ;
#10487=VECTOR ( 'NONE', #18045, 1000.000000000000114 ) ;
#10528=CARTESIAN_POINT ( 'NONE',  ( 0.1285714285714296967, 0.000000000000000000, -5.998622290806041590 ) ) ;
#10533=CARTESIAN_POINT ( 'NONE',  ( 5.284365508485809215, -1.088618427183434934, -2.393569053917001810 ) ) ;
#10534=VECTOR ( 'NONE', #36152, 1000.000000000000000 ) ;
#10546=EDGE_CURVE ( 'NONE', #1529, #37474, #36263, .T. ) ;
#10567=AXIS2_PLACEMENT_3D ( 'NONE', #47579, #18040, #30565 ) ;
#10581=AXIS2_PLACEMENT_3D ( 'NONE', #35796, #18174, #5413 ) ;
#10582=CARTESIAN_POINT ( 'NONE',  ( -66.92263959938523499, -11.38200647523100528, 3.427396607173184062 ) ) ;
#10586=CARTESIAN_POINT ( 'NONE',  ( -67.65221793698312069, 2.688821387764050996E-14, -7.239294561904388026 ) ) ;
#10599=CARTESIAN_POINT ( 'NONE',  ( -66.30127701227512205, 2.000000000000023093, -5.120420914815960955 ) ) ;
#10623=ORIENTED_EDGE ( 'NONE', *, *, #1008, .T. ) ;
#10672=CARTESIAN_POINT ( 'NONE',  ( 5.558065546916891364, 8.867787166497208620E-06, 2.260478567416572826 ) ) ;
#10708=VERTEX_POINT ( 'NONE', #18385 ) ;
#10714=EDGE_CURVE ( 'NONE', #27821, #10380, #32812, .T. ) ;
#10717=ORIENTED_EDGE ( 'NONE', *, *, #49818, .F. ) ;
#10752=CARTESIAN_POINT ( 'NONE',  ( -68.64979563745795588, -9.566959495664058011, -7.934121704141916531 ) ) ;
#10755=ORIENTED_EDGE ( 'NONE', *, *, #19561, .F. ) ;
#10771=CARTESIAN_POINT ( 'NONE',  ( -57.29829478218162109, -10.27834239552269935, 3.000000000000005773 ) ) ;
#10817=STYLED_ITEM ( 'NONE', ( #21608 ), #3559 ) ;
#10833=CARTESIAN_POINT ( 'NONE',  ( -67.69827580336652773, -11.47095193942022995, 5.359670781636989290 ) ) ;
#10837=CARTESIAN_POINT ( 'NONE',  ( -67.81784386561373879, -0.6013392113702856756, -4.340774506266853905 ) ) ;
#10890=ADVANCED_FACE ( 'NONE', ( #49340 ), #48673, .F. ) ;
#10905=CARTESIAN_POINT ( 'NONE',  ( -67.40301992698960021, 2.000000000000002220, -2.652841686095984031 ) ) ;
#10919=CARTESIAN_POINT ( 'NONE',  ( 5.592372708928878389, -1.049503284171714013, -2.322659989241096845 ) ) ;
#10962=CARTESIAN_POINT ( 'NONE',  ( 0.1285714285714296967, 2.000000000000000000, 5.998622290806041590 ) ) ;
#11001=CARTESIAN_POINT ( 'NONE',  ( -66.02636694011434315, -9.266119898376031117, 1.786740587087118470 ) ) ;
#11026=CARTESIAN_POINT ( 'NONE',  ( 4.848100717410754434, 0.000000000000000000, -2.061810099490656079 ) ) ;
#11073=DIRECTION ( 'NONE',  ( 0.9997703818010067467, -0.000000000000000000, -0.02142857142857158143 ) ) ;
#11101=CARTESIAN_POINT ( 'NONE',  ( -67.40002305061796051, -5.356753701341379876E-12, -4.884162593219334880 ) ) ;
#11112=DIRECTION ( 'NONE',  ( 0.9932609354084158682, 0.1139014070068027351, -0.02142857142857155367 ) ) ;
#11159=CARTESIAN_POINT ( 'NONE',  ( 0.09621548157177267635, -1.683565401097097292, -3.964956190634383833E-16 ) ) ;
#11244=ORIENTED_EDGE ( 'NONE', *, *, #14063, .T. ) ;
#11279=CARTESIAN_POINT ( 'NONE',  ( -69.05674355170637568, -0.2656369956482378947, 7.481505251583919325 ) ) ;
#11289=CARTESIAN_POINT ( 'NONE',  ( -65.57807222826096449, -9.214712059194194893, -3.769581895395211379 ) ) ;
#11300=AXIS2_PLACEMENT_3D ( 'NONE', #6390, #40756, #15726 ) ;
#11336=CARTESIAN_POINT ( 'NONE',  ( 0.4518049228021099872, -3.655895688227116747, -5.998622290806042479 ) ) ;
#11345=VERTEX_POINT ( 'NONE', #33363 ) ;
#11394=( NAMED_UNIT ( * ) SI_UNIT ( $, .STERADIAN. ) SOLID_ANGLE_UNIT ( ) );
#11397=CARTESIAN_POINT ( 'NONE',  ( -66.73536025066610478, -1.070822993085610700E-11, -2.844731389951958622 ) ) ;
#11410=CARTESIAN_POINT ( 'NONE',  ( -58.00000000000000711, 2.000000000000000000, -2.999999999999994227 ) ) ;
#11486=ORIENTED_EDGE ( 'NONE', *, *, #13925, .T. ) ;
#11548=EDGE_CURVE ( 'NONE', #19068, #4538, #48098, .T. ) ;
#11582=CARTESIAN_POINT ( 'NONE',  ( -64.81968247311633036, -11.14085154100604669, 2.608662443145389087 ) ) ;
#11585=CARTESIAN_POINT ( 'NONE',  ( -67.83510688862511984, -9.473535711987191021, 6.778377825370747622 ) ) ;
#11590=ORIENTED_EDGE ( 'NONE', *, *, #10546, .T. ) ;
#11631=DIRECTION ( 'NONE',  ( -0.9997703818010067467, 0.000000000000000000, -0.02142857142857158143 ) ) ;
#11643=CARTESIAN_POINT ( 'NONE',  ( -65.81867386097172812, -9.242302859876021515, 4.515874129472566167 ) ) ;
#11671=CARTESIAN_POINT ( 'NONE',  ( -67.50471298836741596, -11.44875527771900714, -8.536061506171076729 ) ) ;
#11678=CARTESIAN_POINT ( 'NONE',  ( 5.128790131151321319, -6.249319155997272723, 2.187078792930187809 ) ) ;
#11713=CARTESIAN_POINT ( 'NONE',  ( 0.000000000000000000, 2.000000000000000000, 0.000000000000000000 ) ) ;
#11727=CARTESIAN_POINT ( 'NONE',  ( -67.59754387994223634, -9.446293363096273765, 7.461800464507162722 ) ) ;
#11728=CARTESIAN_POINT ( 'NONE',  ( -68.69403907479946270, 0.1329702639046175805, 5.527125342194959323 ) ) ;
#11741=CARTESIAN_POINT ( 'NONE',  ( -70.97773365363613607, 1.999999999999998224, -8.809708619959527809 ) ) ;
#11765=VERTEX_POINT ( 'NONE', #10771 ) ;
#11838=CARTESIAN_POINT ( 'NONE',  ( -67.65173211775538675, -9.452507356115830817, 6.473804834638488437 ) ) ;
#11849=FACE_OUTER_BOUND ( 'NONE', #20354, .T. ) ;
#11884=DIRECTION ( 'NONE',  ( -0.1139275668495183524, 0.9934890585767659488, 4.694855797473117491E-16 ) ) ;
#11933=CARTESIAN_POINT ( 'NONE',  ( -66.92698279747418155, 1.734723475976807094E-15, 5.887047890942916695 ) ) ;
#11994=CARTESIAN_POINT ( 'NONE',  ( -67.39275645683859750, 0.1329239778084786161, -1.367274824955979851 ) ) ;
#12012=CARTESIAN_POINT ( 'NONE',  ( -67.68419632946157094, 1.999999999973934850, -3.410887992491007825 ) ) ;
#12015=CARTESIAN_POINT ( 'NONE',  ( -67.90158791901538393, -0.6013636351494499044, -4.591303796237528267 ) ) ;
#12016=CARTESIAN_POINT ( 'NONE',  ( 5.515120863165694942, -1.062156740595928683, 2.500028430129012325 ) ) ;
#12035=ORIENTED_EDGE ( 'NONE', *, *, #11548, .F. ) ;
#12103=DIRECTION ( 'NONE',  ( -0.1139275668495183524, 0.9934890585767659488, 4.694855797473114533E-16 ) ) ;
#12126=CARTESIAN_POINT ( 'NONE',  ( -65.94712367639533568, -9.257032740197443488, 4.837977870786231982 ) ) ;
#12129=CARTESIAN_POINT ( 'NONE',  ( -68.86155229709348191, -10.74924159303523830, -7.491897809418652798 ) ) ;
#12226=CARTESIAN_POINT ( 'NONE',  ( -69.27886756364613063, -9.773082162198893030, -7.306024462451856216 ) ) ;
#12233=DIRECTION ( 'NONE',  ( 0.9090593428863090741, 0.000000000000000000, 0.4166666666666674623 ) ) ;
#12323=CARTESIAN_POINT ( 'NONE',  ( -69.53817124046049969, 0.1329910790360524786, -6.894786738958806005 ) ) ;
#12328=CARTESIAN_POINT ( 'NONE',  ( -67.03776378471746966, -0.6009246745546259483, 0.6758588499069816402 ) ) ;
#12369=EDGE_LOOP ( 'NONE', ( #42617, #1226 ) ) ;
#12407=CARTESIAN_POINT ( 'NONE',  ( 5.681647518099910421, -6.217723448642447082, -2.166220689508504549 ) ) ;
#12427=VERTEX_POINT ( 'NONE', #23219 ) ;
#12527=CARTESIAN_POINT ( 'NONE',  ( -67.66270444019232855, -5.290906601729261638E-14, 7.224227263221078665 ) ) ;
#12600=CARTESIAN_POINT ( 'NONE',  ( -65.33958530469845982, 1.999999999999986233, 0.8132580553645364363 ) ) ;
#12603=CARTESIAN_POINT ( 'NONE',  ( -68.18363897928762185, -0.6010854823554140358, 5.199837068550145602 ) ) ;
#12626=APPLICATION_CONTEXT ( 'automotive_design' ) ;
#12696=CARTESIAN_POINT ( 'NONE',  ( -66.39152944734560435, -11.32110184138706721, -6.891906871564133397 ) ) ;
#12713=CARTESIAN_POINT ( 'NONE',  ( -68.13729736978412177, -4.474875060344467114E-15, -7.461798308327053597 ) ) ;
#12749=ORIENTED_EDGE ( 'NONE', *, *, #44255, .T. ) ;
#12789=CARTESIAN_POINT ( 'NONE',  ( -67.68550200468050093, 4.300705092652487184E-12, 5.522897687430759817 ) ) ;
#12793=B_SPLINE_CURVE_WITH_KNOTS ( 'NONE', 3,
 ( #20930, #12713, #38255, #42533, #24935, #16688 ),
 .UNSPECIFIED., .F., .F.,
 ( 4, 2, 4 ),
 ( 1.406724837889273990E-17, 0.0009531277170912122671, 0.001906255434182410440 ),
 .UNSPECIFIED. ) ;
#12819=ORIENTED_EDGE ( 'NONE', *, *, #34482, .F. ) ;
#12857=DIRECTION ( 'NONE',  ( -0.000000000000000000, -1.000000000000000000, -0.000000000000000000 ) ) ;
#12868=CARTESIAN_POINT ( 'NONE',  ( -69.43683623637159030, 1.999999999998648192, -6.967005367353809042 ) ) ;
#12903=CARTESIAN_POINT ( 'NONE',  ( -69.59775774058348929, -0.6007421665236040154, 7.493101075386322307 ) ) ;
#13025=CARTESIAN_POINT ( 'NONE',  ( -69.22435732763806016, -9.766609940218463848, 7.235198260161168626 ) ) ;
#13029=EDGE_CURVE ( 'NONE', #994, #13853, #28801, .T. ) ;
#13037=EDGE_LOOP ( 'NONE', ( #47260, #1979 ) ) ;
#13041=ORIENTED_EDGE ( 'NONE', *, *, #50262, .F. ) ;
#13044=DIRECTION ( 'NONE',  ( 0.05705673239519650636, -0.9983709377222390602, -2.351258244848514932E-16 ) ) ;
#13064=ORIENTED_EDGE ( 'NONE', *, *, #23025, .T. ) ;
#13134=VERTEX_POINT ( 'NONE', #14482 ) ;
#13147=LINE ( 'NONE', #42664, #38879 ) ;
#13156=CARTESIAN_POINT ( 'NONE',  ( -68.04115265051312633, 1.999999999990856203, 4.403654818465982501 ) ) ;
#13230=CYLINDRICAL_SURFACE ( 'NONE', #10567, 6.000000000000001776 ) ;
#13252=ORIENTED_EDGE ( 'NONE', *, *, #23040, .T. ) ;
#13269=CARTESIAN_POINT ( 'NONE',  ( 4.902479726011972794, 0.000000000000000000, -2.247047898273223598 ) ) ;
#13342=DIRECTION ( 'NONE',  ( -0.05705673239519651330, 0.9983709377222391712, 2.351258244848514932E-16 ) ) ;
#13373=DIRECTION ( 'NONE',  ( 0.000000000000000000, 0.000000000000000000, 1.000000000000000000 ) ) ;
#13461=CARTESIAN_POINT ( 'NONE',  ( -69.66347483736342383, -8.676648739292067702, -7.503912900124009688 ) ) ;
#13556=CARTESIAN_POINT ( 'NONE',  ( 5.519498461031219882, -1.055017498708691992, -2.502222228327667608 ) ) ;
#13579=CARTESIAN_POINT ( 'NONE',  ( -68.13541175005632056, -9.641814632260039986, 5.527125342194959323 ) ) ;
#13580=CARTESIAN_POINT ( 'NONE',  ( 0.1285714285714289751, 0.000000000000000000, 5.998622290806042479 ) ) ;
#13662=VERTEX_POINT ( 'NONE', #6451 ) ;
#13704=CARTESIAN_POINT ( 'NONE',  ( -67.50702643244157741, 2.000000000000000000, -7.448289400635801805 ) ) ;
#13769=LINE ( 'NONE', #433, #10487 ) ;
#13815=CARTESIAN_POINT ( 'NONE',  ( 0.4518049228021099872, -3.655895688227116747, -5.998622290806042479 ) ) ;
#13823=FACE_OUTER_BOUND ( 'NONE', #14172, .T. ) ;
#13853=VERTEX_POINT ( 'NONE', #52120 ) ;
#13860=VERTEX_POINT ( 'NONE', #48416 ) ;
#13916=DIRECTION ( 'NONE',  ( -0.02142857142857158143, 0.000000000000000000, -0.9997703818010067467 ) ) ;
#13925=EDGE_CURVE ( 'NONE', #55181, #29912, #13769, .T. ) ;
#13957=B_SPLINE_CURVE_WITH_KNOTS ( 'NONE', 3,
 ( #14483, #19277, #2235, #6250, #22997, #40316, #40868, #27247, #53642, #1689, #14749, #36083 ),
 .UNSPECIFIED., .F., .F.,
 ( 4, 2, 2, 2, 2, 4 ),
 ( 0.07980989636644560126, 0.1159099261691615840, 0.2318198523383231402, 0.4636397046766463914, 0.6954595570149695316, 0.9272794093314227215 ),
 .UNSPECIFIED. ) ;
#13977=CARTESIAN_POINT ( 'NONE',  ( 4.912750499197525045, -1.131233082521085231, 2.061810099490657411 ) ) ;
#13994=CARTESIAN_POINT ( 'NONE',  ( -65.38649145641349492, 1.999999999999980016, 1.314563741827306620 ) ) ;
#14063=EDGE_CURVE ( 'NONE', #13134, #33308, #15198, .T. ) ;
#14068=CIRCLE ( 'NONE', #4091, 3.000000000000001332 ) ;
#14097=EDGE_CURVE ( 'NONE', #22349, #25311, #40600, .T. ) ;
#14104=ORIENTED_EDGE ( 'NONE', *, *, #16120, .T. ) ;
#14172=EDGE_LOOP ( 'NONE', ( #2876, #253, #13252 ) ) ;
#14282=CARTESIAN_POINT ( 'NONE',  ( -67.07589540981676635, -9.520291518544306442, -2.709928232729476694 ) ) ;
#14354=CARTESIAN_POINT ( 'NONE',  ( -67.32216720457572023, -8.809864171621468287, 4.273291358077422331 ) ) ;
#14426=CARTESIAN_POINT ( 'NONE',  ( -66.31760998578604926, 3.414724497084775940E-15, -0.1846293804859178989 ) ) ;
#14445=EDGE_CURVE ( 'NONE', #5292, #36795, #49753, .T. ) ;
#14482=CARTESIAN_POINT ( 'NONE',  ( 5.057731014323089802, -1.114607557371862567, -2.289010529401726224 ) ) ;
#14483=CARTESIAN_POINT ( 'NONE',  ( -70.10219403106212610, -1.000000000000000666, -7.503912900124007912 ) ) ;
#14492=PLANE ( 'NONE',  #10581 ) ;
#14508=EDGE_CURVE ( 'NONE', #44205, #29912, #50004, .T. ) ;
#14514=CARTESIAN_POINT ( 'NONE',  ( 5.618093942130458096, -1.050357310661657939, 2.260478214906367800 ) ) ;
#14519=EDGE_CURVE ( 'NONE', #45407, #39622, #51133, .T. ) ;
#14534=CARTESIAN_POINT ( 'NONE',  ( -66.74269294525370810, -11.36137123595008269, -2.738438791722735743 ) ) ;
#14539=CARTESIAN_POINT ( 'NONE',  ( -66.50839368374572302, 1.729872094282792178E-11, -1.425848428484772112 ) ) ;
#14590=CARTESIAN_POINT ( 'NONE',  ( 4.912750499197525045, -1.131233082521085231, 2.061810099490657411 ) ) ;
#14621=FACE_BOUND ( 'NONE', #13037, .T. ) ;
#14624=LINE ( 'NONE', #41839, #28351 ) ;
#14680=CARTESIAN_POINT ( 'NONE',  ( -69.45075675106602375, 5.509042946743876566E-16, 8.251517284182453338 ) ) ;
#14749=CARTESIAN_POINT ( 'NONE',  ( -69.18604761972393646, -0.9999999999995238253, 6.394134653913046584 ) ) ;
#14752=ADVANCED_FACE ( 'NONE', ( #44863 ), #14492, .F. ) ;
#14776=( BOUNDED_CURVE ( )  B_SPLINE_CURVE ( 3, ( #20669, #17231, #51864, #38541 ),
 .UNSPECIFIED., .F., .F. ) 
 B_SPLINE_CURVE_WITH_KNOTS ( ( 4, 4 ),
 ( 5.898329122556067894, 6.668041491803113452 ),
 .UNSPECIFIED. ) 
 CURVE ( )  GEOMETRIC_REPRESENTATION_ITEM ( )  RATIONAL_B_SPLINE_CURVE ( ( 1.000000000000000000, 0.9512349561781446861, 0.9512349561781446861, 1.000000000000000000 ) ) 
 REPRESENTATION_ITEM ( '' )  );
#14780=CARTESIAN_POINT ( 'NONE',  ( -69.59775774058348929, -0.6007421665236040154, 7.493101075386322307 ) ) ;
#14791=EDGE_LOOP ( 'NONE', ( #23787, #45872, #34345, #13064 ) ) ;
#14814=CARTESIAN_POINT ( 'NONE',  ( -65.69817947455537421, -11.24159248525151078, 5.466724623770281788 ) ) ;
#14818=CARTESIAN_POINT ( 'NONE',  ( -65.72289477776887168, -3.035766082959412415E-14, 1.903866651545371269 ) ) ;
#14832=CARTESIAN_POINT ( 'NONE',  ( 0.000000000000000000, 2.000000000000000000, -2.125000000000000000 ) ) ;
#14840=ORIENTED_EDGE ( 'NONE', *, *, #30580, .F. ) ;
#14875=CARTESIAN_POINT ( 'NONE',  ( -57.52614991588065152, -8.291364278369165675, -2.999999999999996003 ) ) ;
#15017=VECTOR ( 'NONE', #28739, 1000.000000000000000 ) ;
#15111=CARTESIAN_POINT ( 'NONE',  ( -66.84206714067370569, -9.493454880241955607, -1.367029069777546457 ) ) ;
#15116=CARTESIAN_POINT ( 'NONE',  ( -69.65753061157268178, -0.6010127178502197021, -7.568661514997570450 ) ) ;
#15118=CARTESIAN_POINT ( 'NONE',  ( 0.09621548157177391147, -1.683565401097097070, -3.964956190634383340E-16 ) ) ;
#15130=( BOUNDED_SURFACE ( )  B_SPLINE_SURFACE ( 3, 2, ( 
 ( #40921, #9994, #2304 ),
 ( #18506, #19640, #23350 ),
 ( #53698, #36385, #6303 ),
 ( #54270, #40669, #35851 ),
 ( #31593, #10833, #49985 ),
 ( #19063, #27044, #14814 ),
 ( #23606, #22767, #32679 ),
 ( #36136, #10582, #49465 ),
 ( #44353, #27894, #45201 ),
 ( #2003, #36971, #5453 ),
 ( #40381, #32141, #45453 ),
 ( #18815, #19340, #53995 ),
 ( #15111, #53174, #32435 ),
 ( #14282, #14534, #53437 ),
 ( #48899, #6567, #23879 ),
 ( #27301, #44615, #5734 ),
 ( #23059, #31849, #49160 ),
 ( #10274, #27598, #44923 ),
 ( #6037, #45735, #34107 ),
 ( #3135, #20164, #15933 ),
 ( #16207, #51118, #25298 ),
 ( #12226, #24438, #11671 ),
 ( #33525, #20750, #50833 ),
 ( #6864, #37499, #7140 ) ),
 .UNSPECIFIED., .F., .F., .F. ) 
 B_SPLINE_SURFACE_WITH_KNOTS ( ( 4, 2, 2, 2, 2, 2, 2, 2, 2, 2, 2, 4 ),
 ( 3, 3 ),
 ( 0.008994972463978564287, 0.01138926720843922921, 0.01258641458066956167, 0.01378356195289989587, 0.01617785669736056253, 0.01857215144182122746, 0.02096644618628189238, 0.02336074093074255731, 0.02575503567520322223, 0.02695218304743355470, 0.02755075673354872440, 0.02814933041966389063 ),
 ( 0.000000000000000000, 1.000000000000000000 ),
 .UNSPECIFIED. ) 
 GEOMETRIC_REPRESENTATION_ITEM ( )  RATIONAL_B_SPLINE_SURFACE ( (
 ( 1.000000000000000000, 0.7302382283600511448, 1.000000000000000000),
 ( 1.000000000000000000, 0.7302057701444357729, 1.000000000000000000),
 ( 1.000000000000000000, 0.7302261543188973691, 1.000000000000000000),
 ( 1.000000000000000000, 0.7302340627759303926, 1.000000000000000000),
 ( 1.000000000000000000, 0.7302358193541355069, 1.000000000000000000),
 ( 1.000000000000000000, 0.7302356584975112641, 1.000000000000000000),
 ( 1.000000000000000000, 0.7302336981016072093, 1.000000000000000000),
 ( 1.000000000000000000, 0.7302244465200464774, 1.000000000000000000),
 ( 1.000000000000000000, 0.7302382397014047788, 1.000000000000000000),
 ( 1.000000000000000000, 0.7302438375889021005, 1.000000000000000000),
 ( 1.000000000000000000, 0.7302379409284335265, 1.000000000000000000),
 ( 1.000000000000000000, 0.7302249128382346521, 1.000000000000000000),
 ( 1.000000000000000000, 0.7302266904902104949, 1.000000000000000000),
 ( 1.000000000000000000, 0.7302305284537528030, 1.000000000000000000),
 ( 1.000000000000000000, 0.7302278475275691960, 1.000000000000000000),
 ( 1.000000000000000000, 0.7302208473896385499, 1.000000000000000000),
 ( 1.000000000000000000, 0.7302205818819856864, 1.000000000000000000),
 ( 1.000000000000000000, 0.7302413824365678874, 1.000000000000000000),
 ( 1.000000000000000000, 0.7302489349981282629, 1.000000000000000000),
 ( 1.000000000000000000, 0.7302381596259744923, 1.000000000000000000),
 ( 1.000000000000000000, 0.7302138215212032879, 1.000000000000000000),
 ( 1.000000000000000000, 0.7302588551347022339, 1.000000000000000000),
 ( 1.000000000000000000, 0.7302821861409102278, 1.000000000000000000),
 ( 1.000000000000000000, 0.7303030204721967511, 1.000000000000000000) ) ) 
 REPRESENTATION_ITEM ( '' )  SURFACE ( )  );
#15198=LINE ( 'NONE', #23434, #24946 ) ;
#15237=DIRECTION ( 'NONE',  ( -0.1139275668495183386, 0.9934890585767658377, 4.694855797473113547E-16 ) ) ;
#15259=CARTESIAN_POINT ( 'NONE',  ( -69.99028037491666510, 0.2761374490229266399, -7.501514206501484594 ) ) ;
#15284=CARTESIAN_POINT ( 'NONE',  ( -67.76121356559087872, -9.465062053996337710, 8.159882300530348687 ) ) ;
#15363=FACE_OUTER_BOUND ( 'NONE', #46248, .T. ) ;
#15367=CARTESIAN_POINT ( 'NONE',  ( -68.75638519912476454, -2.100476156393307137E-11, -7.380886937888696764 ) ) ;
#15406=DIRECTION ( 'NONE',  ( 0.000000000000000000, 0.000000000000000000, 1.000000000000000000 ) ) ;
#15518=ORIENTED_EDGE ( 'NONE', *, *, #4511, .F. ) ;
#15532=CARTESIAN_POINT ( 'NONE',  ( -65.19876137812605066, -9.171214889434388340, 1.903866651539666943 ) ) ;
#15548=CARTESIAN_POINT ( 'NONE',  ( -69.11683642851026832, -9.015837829197110409, 7.493101075386320531 ) ) ;
#15553=DIRECTION ( 'NONE',  ( -0.1139275668495183524, 0.9934890585767659488, 4.694855797473114533E-16 ) ) ;
#15609=ORIENTED_EDGE ( 'NONE', *, *, #5465, .F. ) ;
#15629=( LENGTH_UNIT ( ) NAMED_UNIT ( * ) SI_UNIT ( .MILLI., .METRE. ) );
#15631=CARTESIAN_POINT ( 'NONE',  ( -66.55592414517043665, -9.044681206892926412E-12, 1.786740587093984534 ) ) ;
#15640=CARTESIAN_POINT ( 'NONE',  ( -58.00000000000000711, 0.000000000000000000, -2.999999999999994227 ) ) ;
#15702=LINE ( 'NONE', #29908, #31419 ) ;
#15722=DIRECTION ( 'NONE',  ( -0.05705673239519651330, 0.9983709377222390602, 2.401210743435858319E-16 ) ) ;
#15725=CARTESIAN_POINT ( 'NONE',  ( 0.09621548157177266247, -1.683565401097097070, -3.964956190634384326E-16 ) ) ;
#15726=DIRECTION ( 'NONE',  ( 0.000000000000000000, -0.000000000000000000, -1.000000000000000000 ) ) ;
#15745=AXIS2_PLACEMENT_3D ( 'NONE', #40050, #299, #31561 ) ;
#15812=EDGE_LOOP ( 'NONE', ( #25964, #9329 ) ) ;
#15823=CARTESIAN_POINT ( 'NONE',  ( -66.38245585351968714, -9.306954111037352817, -3.536654368697047968 ) ) ;
#15832=EDGE_CURVE ( 'NONE', #18640, #3029, #20031, .T. ) ;
#15840=CARTESIAN_POINT ( 'NONE',  ( 4.912750499197526821, -1.131233082521083455, -2.061810099490656079 ) ) ;
#15847=ORIENTED_EDGE ( 'NONE', *, *, #3224, .F. ) ;
#15879=FACE_BOUND ( 'NONE', #2018, .T. ) ;
#15926=AXIS2_PLACEMENT_3D ( 'NONE', #53338, #22401, #48494 ) ;
#15933=CARTESIAN_POINT ( 'NONE',  ( -67.14664173531406277, -11.40769374184509388, -8.053057903409269969 ) ) ;
#15981=ADVANCED_FACE ( 'NONE', ( #18794 ), #35827, .F. ) ;
#16004=CARTESIAN_POINT ( 'NONE',  ( -67.62088067883519216, 0.1329945644841871721, 2.681528892132510222 ) ) ;
#16016=ORIENTED_EDGE ( 'NONE', *, *, #54015, .T. ) ;
#16017=CARTESIAN_POINT ( 'NONE',  ( -70.45024891871291572, 2.000000000000000000, 8.217082732571151737 ) ) ;
#16018=B_SPLINE_CURVE_WITH_KNOTS ( 'NONE', 3,
 ( #35618, #23663, #49796, #50635, #2369, #20231, #11727, #40984 ),
 .UNSPECIFIED., .F., .F.,
 ( 4, 2, 2, 4 ),
 ( 4.827458356132498828E-16, 0.0004770940840306632427, 0.0009541881680608437985, 0.001908376336121245459 ),
 .UNSPECIFIED. ) ;
#16029=CARTESIAN_POINT ( 'NONE',  ( 5.585384566839274534, -1.054099306315943396, 2.341018106606942428 ) ) ;
#16118=CARTESIAN_POINT ( 'NONE',  ( -64.95503971932161846, -11.15637352545318706, 3.244935472806012022 ) ) ;
#16120=EDGE_CURVE ( 'NONE', #22349, #32717, #3502, .T. ) ;
#16122=CARTESIAN_POINT ( 'NONE',  ( -66.67188136048933700, -8.735183455216070314, -1.700609907707529400 ) ) ;
#16207=CARTESIAN_POINT ( 'NONE',  ( -69.07439616956314410, -9.749369762244352700, -7.034467916848615943 ) ) ;
#16254=( BOUNDED_CURVE ( )  B_SPLINE_CURVE ( 3, ( #1857, #27429, #27739, #44758 ),
 .UNSPECIFIED., .F., .F. ) 
 B_SPLINE_CURVE_WITH_KNOTS ( ( 4, 4 ),
 ( 1.140403016137406356, 2.754752525938840790 ),
 .UNSPECIFIED. ) 
 CURVE ( )  GEOMETRIC_REPRESENTATION_ITEM ( )  RATIONAL_B_SPLINE_CURVE ( ( 1.000000000000000000, 0.7943613114863616875, 0.7943613114863616875, 1.000000000000000000 ) ) 
 REPRESENTATION_ITEM ( '' )  );
#16264=CARTESIAN_POINT ( 'NONE',  ( -68.25801324219597177, 0.1329745449598424278, 4.605078063924990417 ) ) ;
#16279=CARTESIAN_POINT ( 'NONE',  ( -67.56998338746467425, 1.999999999999990452, 7.586268967162788535 ) ) ;
#16323=EDGE_CURVE ( 'NONE', #13662, #53459, #20896, .T. ) ;
#16329=VERTEX_POINT ( 'NONE', #53552 ) ;
#16356=VERTEX_POINT ( 'NONE', #36511 ) ;
#16375=AXIS2_PLACEMENT_3D ( 'NONE', #55124, #25563, #41753 ) ;
#16376=CARTESIAN_POINT ( 'NONE',  ( -65.38876380835138491, -9.193003266854505640, -3.032880804691990395 ) ) ;
#16378=CARTESIAN_POINT ( 'NONE',  ( -69.23151552270924469, -10.31681141643477773, -7.498719848001563548 ) ) ;
#16479=AXIS2_PLACEMENT_3D ( 'NONE', #12407, #9237, #29735 ) ;
#16523=VERTEX_POINT ( 'NONE', #25687 ) ;
#16556=CARTESIAN_POINT ( 'NONE',  ( -68.39906907640694556, 2.000000000000000000, -8.694190345976133827 ) ) ;
#16584=EDGE_LOOP ( 'NONE', ( #33446, #13041, #52750, #21032 ) ) ;
#16643=CARTESIAN_POINT ( 'NONE',  ( -69.20821692254106949, -9.630996011957124736, 8.593930712158170948 ) ) ;
#16688=CARTESIAN_POINT ( 'NONE',  ( -69.59783862807636012, -0.6008070088998225255, -7.493102809087827332 ) ) ;
#16772=( LENGTH_UNIT ( ) NAMED_UNIT ( * ) SI_UNIT ( .MILLI., .METRE. ) );
#16864=CARTESIAN_POINT ( 'NONE',  ( -68.44534682279325466, 1.999999999991179056, -5.350280945793637777 ) ) ;
#16868=CARTESIAN_POINT ( 'NONE',  ( -68.17347556353657012, -0.6006513931709031029, -5.215119943113104561 ) ) ;
#16893=ORIENTED_EDGE ( 'NONE', *, *, #38278, .F. ) ;
#16942=FACE_OUTER_BOUND ( 'NONE', #33704, .T. ) ;
#16949=CARTESIAN_POINT ( 'NONE',  ( -65.78960443026792859, -9.238969346053028886, -0.1846293804859200915 ) ) ;
#16970=CARTESIAN_POINT ( 'NONE',  ( -64.58804046960723610, -11.11428817866989149, -1.324960789524878946 ) ) ;
#17072=ADVANCED_FACE ( 'NONE', ( #46635 ), #21909, .F. ) ;
#17138=CARTESIAN_POINT ( 'NONE',  ( -67.33297928875471428, 0.1329136931077638251, -0.6892805327783358971 ) ) ;
#17227=ORIENTED_EDGE ( 'NONE', *, *, #42339, .T. ) ;
#17231=CARTESIAN_POINT ( 'NONE',  ( 5.446213544912835935, -1.070058632457643766, -0.6896135826588382089 ) ) ;
#17243=CARTESIAN_POINT ( 'NONE',  ( -68.01236371044051054, -8.487308885305189676, 5.059064008999122564 ) ) ;
#17256=DIRECTION ( 'NONE',  ( 0.000000000000000000, 0.000000000000000000, -1.000000000000000000 ) ) ;
#17296=CARTESIAN_POINT ( 'NONE',  ( -70.10219403106212610, -1.000000000000000666, -7.503912900124007912 ) ) ;
#17301=ORIENTED_EDGE ( 'NONE', *, *, #30444, .F. ) ;
#17316=SURFACE_STYLE_FILL_AREA ( #42881 ) ;
#17329=B_SPLINE_SURFACE_WITH_KNOTS ( 'NONE', 1, 3, ( 
 ( #27765, #44492, #36276, #22650, #18103, #32005, #35715, #18958, #45088, #36023, #5601, #31472, #27461, #22925 ),
 ( #40245, #5899, #48788, #1336, #53329, #18374, #23225, #14426, #35427, #1632, #53574, #31734, #14680, #49038 ) ),
 .UNSPECIFIED., .F., .F., .F.,
 ( 2, 2 ),
 ( 4, 2, 2, 2, 2, 2, 4 ),
 ( 0.000000000000000000, 1.000000000000000000 ),
 ( 0.000000000000000000, 0.1159099261691615840, 0.2318198523383231680, 0.4636397046766463359, 0.6954595570149695316, 0.9272794093532926718, 1.000000000000000000 ),
 .UNSPECIFIED. ) ;
#17331=APPLICATION_CONTEXT ( 'automotive_design' ) ;
#17360=DIRECTION ( 'NONE',  ( 0.000000000000000000, 0.000000000000000000, 1.000000000000000000 ) ) ;
#17391=ADVANCED_FACE ( 'NONE', ( #24698 ), #20999, .T. ) ;
#17392=DIRECTION ( 'NONE',  ( 0.000000000000000000, 5.782411586589354681E-16, -1.000000000000000000 ) ) ;
#17397=CARTESIAN_POINT ( 'NONE',  ( -66.30048190469359781, 1.999999999999976685, 5.092367036307550165 ) ) ;
#17419=VERTEX_POINT ( 'NONE', #17296 ) ;
#17455=CARTESIAN_POINT ( 'NONE',  ( 0.09621548157177391147, -1.683565401097097070, -3.964956190634383340E-16 ) ) ;
#17485=CARTESIAN_POINT ( 'NONE',  ( -57.29829478218162109, -10.27834239552269757, 4.211285351864063224E-15 ) ) ;
#17569=ORIENTED_EDGE ( 'NONE', *, *, #10192, .F. ) ;
#17579=CARTESIAN_POINT ( 'NONE',  ( -66.34585003275293502, 4.336808689942017736E-15, -4.508581566067807245 ) ) ;
#17598=ORIENTED_EDGE ( 'NONE', *, *, #55504, .F. ) ;
#17781=CARTESIAN_POINT ( 'NONE',  ( 0.3240706152708093812, -3.670543518250628967, -1.335466778558061241E-15 ) ) ;
#17809=CARTESIAN_POINT ( 'NONE',  ( 4.848100717410754434, 0.000000000000000000, -2.061810099490656079 ) ) ;
#17834=VERTEX_POINT ( 'NONE', #15840 ) ;
#17920=CARTESIAN_POINT ( 'NONE',  ( 5.577510371788089394, -6.223674869166635482, -2.393421119419574250 ) ) ;
#17948=ORIENTED_EDGE ( 'NONE', *, *, #14097, .T. ) ;
#17962=CARTESIAN_POINT ( 'NONE',  ( -70.00259797851279586, 0.1329035588801656675, 7.501778215771297553 ) ) ;
#18006=CARTESIAN_POINT ( 'NONE',  ( -67.08542992444135677, -8.381013491352103273, 2.158836163547856124 ) ) ;
#18040=DIRECTION ( 'NONE',  ( -0.000000000000000000, -1.000000000000000000, -0.000000000000000000 ) ) ;
#18045=DIRECTION ( 'NONE',  ( -0.1139275668495183386, 0.9934890585767658377, 4.694855797473113547E-16 ) ) ;
#18047=EDGE_CURVE ( 'NONE', #27104, #32512, #29995, .T. ) ;
#18103=CARTESIAN_POINT ( 'NONE',  ( -68.93342745996714882, -0.9999999999999983347, -5.847034362371242189 ) ) ;
#18168=CARTESIAN_POINT ( 'NONE',  ( 2.602374448188125350E-16, 0.000000000000000000, 2.125000000000000000 ) ) ;
#18169=CARTESIAN_POINT ( 'NONE',  ( 4.912750499197526821, -1.131233082521083455, -2.061810099490656079 ) ) ;
#18172=AXIS2_PLACEMENT_3D ( 'NONE', #11678, #42607, #12233 ) ;
#18174=DIRECTION ( 'NONE',  ( -0.02142857142857158143, 0.000000000000000000, 0.9997703818010067467 ) ) ;
#18184=CARTESIAN_POINT ( 'NONE',  ( 5.454592090961233097, -6.230699628392518008, 2.061810099490656079 ) ) ;
#18188=ORIENTED_EDGE ( 'NONE', *, *, #34591, .T. ) ;
#18307=AXIS2_PLACEMENT_3D ( 'NONE', #15725, #20571, #54091 ) ;
#18326=EDGE_LOOP ( 'NONE', ( #42585, #6927, #22268, #52642, #53801, #50329, #30146 ) ) ;
#18374=CARTESIAN_POINT ( 'NONE',  ( -67.34283022341989522, -3.900800535205241593E-15, -5.009371237985868142 ) ) ;
#18385=CARTESIAN_POINT ( 'NONE',  ( -67.27731269685068582, -9.409571107119717226, -7.454891809856700746 ) ) ;
#18396=ORIENTED_EDGE ( 'NONE', *, *, #51491, .F. ) ;
#18403=ORIENTED_EDGE ( 'NONE', *, *, #2315, .F. ) ;
#18417=VERTEX_POINT ( 'NONE', #39175 ) ;
#18442=DIRECTION ( 'NONE',  ( -0.1139275668495183524, 0.9934890585767659488, 4.694855797473114533E-16 ) ) ;
#18480=AXIS2_PLACEMENT_3D ( 'NONE', #54755, #32898, #24951 ) ;
#18506=CARTESIAN_POINT ( 'NONE',  ( -69.06652772757389869, -9.747969413217129286, 7.053755868282013175 ) ) ;
#18536=CARTESIAN_POINT ( 'NONE',  ( -69.61318730843225921, -8.922530380692753837, -7.503442492476276371 ) ) ;
#18547=ORIENTED_EDGE ( 'NONE', *, *, #34203, .T. ) ;
#18560=CARTESIAN_POINT ( 'NONE',  ( 4.848100717410752658, 0.000000000000000000, 2.061810099490657411 ) ) ;
#18561=CARTESIAN_POINT ( 'NONE',  ( 5.809281049934954311, -6.210429213608743559, -2.500000000000000444 ) ) ;
#18594=CARTESIAN_POINT ( 'NONE',  ( -66.62599605097206279, -8.730077326369423574, -1.335442097082736534 ) ) ;
#18640=VERTEX_POINT ( 'NONE', #30934 ) ;
#18664=LINE ( 'NONE', #40229, #55947 ) ;
#18794=FACE_OUTER_BOUND ( 'NONE', #20443, .T. ) ;
#18808=CARTESIAN_POINT ( 'NONE',  ( -69.87053270868739219, 0.6920041563027308218, 7.498947595741738859 ) ) ;
#18815=CARTESIAN_POINT ( 'NONE',  ( -66.78322018952341921, -9.486696200041539129, -0.6892805327663855675 ) ) ;
#18819=CARTESIAN_POINT ( 'NONE',  ( -67.81219270629397045, -0.6009186479185966157, 4.328853820094372473 ) ) ;
#18828=CARTESIAN_POINT ( 'NONE',  ( -68.52750228004174460, 2.000000000000000000, -8.849861037685109011 ) ) ;
#18830=ORIENTED_EDGE ( 'NONE', *, *, #14508, .T. ) ;
#18837=CARTESIAN_POINT ( 'NONE',  ( -69.56291444385804823, -9.168415021912489138, -7.502972407220386053 ) ) ;
#18871=SURFACE_SIDE_STYLE ('',( #54055 ) ) ;
#18888=CARTESIAN_POINT ( 'NONE',  ( -67.71196402477201559, -8.854389638963908737, 5.199837068550139385 ) ) ;
#18958=CARTESIAN_POINT ( 'NONE',  ( -67.32595136268157887, -0.9999999999999978906, 0.5932824550257459473 ) ) ;
#18974=ORIENTED_EDGE ( 'NONE', *, *, #5465, .T. ) ;
#19044=CARTESIAN_POINT ( 'NONE',  ( 5.385059872733034325, 0.000000000000000000, -0.6896135826588374318 ) ) ;
#19063=CARTESIAN_POINT ( 'NONE',  ( -67.73318103894531816, -9.595695390205156272, 4.678579668398631597 ) ) ;
#19067=CARTESIAN_POINT ( 'NONE',  ( -67.09318657654290519, -0.6008575946992210648, -1.359962337613763950 ) ) ;
#19068=VERTEX_POINT ( 'NONE', #18560 ) ;
#19076=( BOUNDED_CURVE ( )  B_SPLINE_CURVE ( 3, ( #6283, #19044, #32416, #19316 ),
 .UNSPECIFIED., .F., .F. ) 
 B_SPLINE_CURVE_WITH_KNOTS ( ( 4, 4 ),
 ( 5.898329122556067894, 6.668041491803113452 ),
 .UNSPECIFIED. ) 
 CURVE ( )  GEOMETRIC_REPRESENTATION_ITEM ( )  RATIONAL_B_SPLINE_CURVE ( ( 1.000000000000000000, 0.9512349561781446861, 0.9512349561781446861, 1.000000000000000000 ) ) 
 REPRESENTATION_ITEM ( '' )  );
#19090=ADVANCED_FACE ( 'NONE', ( #44394 ), #689, .F. ) ;
#19114=DIRECTION ( 'NONE',  ( 0.000000000000000000, 1.000000000000000000, 0.000000000000000000 ) ) ;
#19121=VECTOR ( 'NONE', #55002, 1000.000000000000114 ) ;
#19134=CARTESIAN_POINT ( 'NONE',  ( -70.53061787018394568, 1.999999999999998224, -8.307376767094712733 ) ) ;
#19173=ORIENTED_EDGE ( 'NONE', *, *, #41113, .F. ) ;
#19177=EDGE_LOOP ( 'NONE', ( #10717, #55281, #26306, #40630, #18403, #39406, #989 ) ) ;
#19212=CARTESIAN_POINT ( 'NONE',  ( -69.85990692124715906, 0.6786957477238007019, -7.498719848001561772 ) ) ;
#19248=EDGE_LOOP ( 'NONE', ( #21802, #34196, #31399, #4013 ) ) ;
#19261=ORIENTED_EDGE ( 'NONE', *, *, #26133, .T. ) ;
#19277=CARTESIAN_POINT ( 'NONE',  ( -69.96872419296560963, -1.000000000000000888, -7.341494710781372390 ) ) ;
#19280=VECTOR ( 'NONE', #28281, 1000.000000000000000 ) ;
#19316=CARTESIAN_POINT ( 'NONE',  ( 4.866417447938704122, 0.000000000000000000, 1.967953638241001002 ) ) ;
#19340=CARTESIAN_POINT ( 'NONE',  ( -66.44695135234023553, -11.32745730419861374, -0.6963329337552829346 ) ) ;
#19344=CARTESIAN_POINT ( 'NONE',  ( -66.47616155185831133, 5.898059818321144121E-14, 4.837977870783337409 ) ) ;
#19362=CARTESIAN_POINT ( 'NONE',  ( -69.43561177275644525, -9.791245164465275153, -7.501782499249458169 ) ) ;
#19437=CARTESIAN_POINT ( 'NONE',  ( 5.343330229674628562, -1.064751996674356826, -2.421220660758175658 ) ) ;
#19480=DIRECTION ( 'NONE',  ( -0.02128905125521653521, -0.002441305003918738115, 0.9997703818010066357 ) ) ;
#19496=DIRECTION ( 'NONE',  ( 0.000000000000000000, 0.000000000000000000, 1.000000000000000000 ) ) ;
#19537=CARTESIAN_POINT ( 'NONE',  ( -67.89698098956576189, -8.875497699457834955, 5.577208301931539935 ) ) ;
#19544=ADVANCED_FACE ( 'NONE', ( #29031 ), #41542, .F. ) ;
#19561=EDGE_CURVE ( 'NONE', #36795, #45113, #30446, .T. ) ;
#19621=AXIS2_PLACEMENT_3D ( 'NONE', #35340, #22287, #21984 ) ;
#19640=CARTESIAN_POINT ( 'NONE',  ( -68.75440753303996644, -11.59206300474163065, 7.127210919649165533 ) ) ;
#19644=CARTESIAN_POINT ( 'NONE',  ( -66.43509620407327532, 1.406259945342289676E-11, 0.3563396980984065432 ) ) ;
#19719=CARTESIAN_POINT ( 'NONE',  ( -69.96913243261153070, 2.000000000000049738, 7.657023247222836559 ) ) ;
#19773=CARTESIAN_POINT ( 'NONE',  ( 4.866417447938705898, 0.000000000000000000, -1.967953638240998337 ) ) ;
#19815=CARTESIAN_POINT ( 'NONE',  ( -66.55921131444038963, -8.722325662721239325, 0.3393403235802882056 ) ) ;
#19832=CARTESIAN_POINT ( 'NONE',  ( 0.3240706152708106025, -3.670543518250628967, -1.335466778558061241E-15 ) ) ;
#19840=EDGE_CURVE ( 'NONE', #37474, #37895, #2820, .T. ) ;
#19870=EDGE_CURVE ( 'NONE', #43429, #33308, #29729, .T. ) ;
#19875=CARTESIAN_POINT ( 'NONE',  ( -65.83373593673759672, -1.561251128379126385E-14, 2.627585852360243113 ) ) ;
#19904=CARTESIAN_POINT ( 'NONE',  ( -67.94414157437554991, -0.6013562474879498021, -4.659789304345617111 ) ) ;
#19915=CARTESIAN_POINT ( 'NONE',  ( 4.994031378522669762, 0.000000000000000000, -2.289010529401725780 ) ) ;
#19924=ORIENTED_EDGE ( 'NONE', *, *, #6156, .T. ) ;
#19991=CARTESIAN_POINT ( 'NONE',  ( -68.51296364132990391, -11.00146576780565866, 7.485090880804395219 ) ) ;
#20019=CARTESIAN_POINT ( 'NONE',  ( 0.000000000000000000, 2.000000000000000000, 0.000000000000000000 ) ) ;
#20031=B_SPLINE_CURVE_WITH_KNOTS ( 'NONE', 1,
 ( #21648, #38960 ),
 .UNSPECIFIED., .F., .F.,
 ( 2, 2 ),
 ( 0.000000000000000000, 0.0006430183911724572481 ),
 .UNSPECIFIED. ) ;
#20058=ORIENTED_EDGE ( 'NONE', *, *, #34482, .T. ) ;
#20070=CARTESIAN_POINT ( 'NONE',  ( -66.85871239793839038, -9.361568451089064880, 4.869406872008419818 ) ) ;
#20087=ORIENTED_EDGE ( 'NONE', *, *, #29162, .F. ) ;
#20137=CARTESIAN_POINT ( 'NONE',  ( -67.45463423721670893, 0.000000000000000000, 6.901237005686192028 ) ) ;
#20164=CARTESIAN_POINT ( 'NONE',  ( -68.66066644775141015, -11.58131332038088246, -6.967005367358785506 ) ) ;
#20231=CARTESIAN_POINT ( 'NONE',  ( -67.91822744485311603, -9.430911930847621250, 7.468591521940118660 ) ) ;
#20234=CARTESIAN_POINT ( 'NONE',  ( -69.58726886377220922, 0.1328949963053452921, 6.962762944060566284 ) ) ;
#20345=ORIENTED_EDGE ( 'NONE', *, *, #32481, .F. ) ;
#20354=EDGE_LOOP ( 'NONE', ( #16016, #11590, #46836, #51120 ) ) ;
#20367=CARTESIAN_POINT ( 'NONE',  ( -66.84374069725500078, -8.754700742360908450, -2.713115426954385789 ) ) ;
#20443=EDGE_LOOP ( 'NONE', ( #38876, #12819, #2587, #54383 ) ) ;
#20562=CARTESIAN_POINT ( 'NONE',  ( -67.80680003470160955, 0.1329109690309568104, 3.391838660566504071 ) ) ;
#20567=CARTESIAN_POINT ( 'NONE',  ( -67.02352122496155573, -0.6009590134347525536, 0.3404743498653474698 ) ) ;
#20569=CARTESIAN_POINT ( 'NONE',  ( 4.993307398318179047, 0.01266810708056629979, -2.289010529401725336 ) ) ;
#20571=DIRECTION ( 'NONE',  ( -0.1139275668495183524, 0.9934890585767659488, 4.694855797473114533E-16 ) ) ;
#20579=CARTESIAN_POINT ( 'NONE',  ( -68.26343194379199986, -11.13167664141646185, 7.480095325092515068 ) ) ;
#20602=CARTESIAN_POINT ( 'NONE',  ( -66.74449147233332269, -11.36157748060019301, 7.448312483692313357 ) ) ;
#20609=DIRECTION ( 'NONE',  ( 0.05705673239519650636, -0.9983709377222390602, -2.351258244848514932E-16 ) ) ;
#20664=CARTESIAN_POINT ( 'NONE',  ( -66.74342152241241877, -11.36145478494482042, -7.448289400635804469 ) ) ;
#20666=ORIENTED_EDGE ( 'NONE', *, *, #30580, .T. ) ;
#20667=CARTESIAN_POINT ( 'NONE',  ( -65.07007842715393053, -9.156458274479485127, -0.3798655365511886539 ) ) ;
#20669=CARTESIAN_POINT ( 'NONE',  ( 4.930947970565946470, -1.129146301979396139, -1.967953638240999670 ) ) ;
#20679=DIRECTION ( 'NONE',  ( 0.000000000000000000, -1.000000000000000000, 0.000000000000000000 ) ) ;
#20683=CARTESIAN_POINT ( 'NONE',  ( -69.97337567751375786, -11.73184720622960953, 8.563005977519212664 ) ) ;
#20704=CARTESIAN_POINT ( 'NONE',  ( 4.912750499197527709, -1.131233082521084343, -2.162384853247615535 ) ) ;
#20750=CARTESIAN_POINT ( 'NONE',  ( -69.07738657957442285, -11.62910036973895878, -7.520604412854629217 ) ) ;
#20821=CARTESIAN_POINT ( 'NONE',  ( -69.63916331601677712, 0.1328488985137141754, -7.034467916851212976 ) ) ;
#20895=CARTESIAN_POINT ( 'NONE',  ( -66.67823795591188230, -9.340872688141725888, 4.722169080041619615 ) ) ;
#20896=( BOUNDED_CURVE ( )  B_SPLINE_CURVE ( 3, ( #5873, #39682, #9575, #36251 ),
 .UNSPECIFIED., .F., .F. ) 
 B_SPLINE_CURVE_WITH_KNOTS ( ( 4, 4 ),
 ( 2.001189637452388759, 3.141592653589797113 ),
 .UNSPECIFIED. ) 
 CURVE ( )  GEOMETRIC_REPRESENTATION_ITEM ( )  RATIONAL_B_SPLINE_CURVE ( ( 1.000000000000000000, 0.8945281452387652266, 0.8945281452387652266, 1.000000000000000000 ) ) 
 REPRESENTATION_ITEM ( '' )  );
#20919=CARTESIAN_POINT ( 'NONE',  ( 5.558065546916891364, 8.867787166497208620E-06, 2.260478567416572826 ) ) ;
#20930=CARTESIAN_POINT ( 'NONE',  ( -67.81506811452879901, 0.000000000000000000, -7.454891809856698970 ) ) ;
#20999=CYLINDRICAL_SURFACE ( 'NONE', #2242, 0.2499999999999998612 ) ;
#21032=ORIENTED_EDGE ( 'NONE', *, *, #24847, .T. ) ;
#21076=CARTESIAN_POINT ( 'NONE',  ( -68.07189119022113744, 1.958909493320992512, 7.460396425438592161 ) ) ;
#21090=CARTESIAN_POINT ( 'NONE',  ( -57.29829478218162109, -10.27834239552269757, 4.211285351864063224E-15 ) ) ;
#21096=CARTESIAN_POINT ( 'NONE',  ( -67.51160766412522207, 1.999999999982350785, 2.764386752165123085 ) ) ;
#21184=CARTESIAN_POINT ( 'NONE',  ( -69.94833770632727976, -8.709315162003530730, 7.852029984319920608 ) ) ;
#21193=VECTOR ( 'NONE', #47383, 1000.000000000000000 ) ;
#21328=CIRCLE ( 'NONE', #8649, 3.000000000000001332 ) ;
#21380=CYLINDRICAL_SURFACE ( 'NONE', #145, 6.000000000000001776 ) ;
#21405=CARTESIAN_POINT ( 'NONE',  ( -67.68741903510353097, 2.000000000018216539, 3.427396607167120912 ) ) ;
#21409=VERTEX_POINT ( 'NONE', #53907 ) ;
#21410=CARTESIAN_POINT ( 'NONE',  ( -67.09379796712988764, -0.6008889714318613740, 1.346828299457901501 ) ) ;
#21433=B_SPLINE_CURVE_WITH_KNOTS ( 'NONE', 3,
 ( #2397, #45831, #50913, #16868, #12015, #51213, #4078, #3778, #34199, #42974, #37594, #20567, #12328, #21410, #3234, #46370, #37888, #25956, #8326, #12603, #3515, #55192, #55755, #38142, #54920, #51510, #29921, #46965 ),
 .UNSPECIFIED., .F., .F.,
 ( 4, 2, 2, 2, 2, 2, 2, 2, 2, 2, 2, 2, 2, 4 ),
 ( 7.806255641895631925E-18, 0.002014507434814110081, 0.004029014869628212356, 0.006043522304442314197, 0.007050776021849361648, 0.008058029739256410834, 0.009065283456663457418, 0.01007253717407050400, 0.01208704460888460064, 0.01309429832629165416, 0.01410155204369870768, 0.01510880576110576468, 0.01561243261980930011, 0.01611605947851283901 ),
 .UNSPECIFIED. ) ;
#21456=VECTOR ( 'NONE', #20609, 1000.000000000000114 ) ;
#21519=CARTESIAN_POINT ( 'NONE',  ( -67.81626209598535127, 0.000000000000000000, 7.454917401049828918 ) ) ;
#21558=LINE ( 'NONE', #38873, #8562 ) ;
#21559=CARTESIAN_POINT ( 'NONE',  ( -67.07240009714290352, -9.519890509981273397, -2.692672496485625455 ) ) ;
#21565=ADVANCED_FACE ( 'NONE', ( #41427 ), #2512, .F. ) ;
#21584=CARTESIAN_POINT ( 'NONE',  ( 5.558065690504402134, 8.867811663421879681E-06, -2.260478214935544017 ) ) ;
#21608=PRESENTATION_STYLE_ASSIGNMENT (( #51958 ) ) ;
#21612=CARTESIAN_POINT ( 'NONE',  ( 5.221828392167458865, 0.000000000000000000, 2.393421119419573806 ) ) ;
#21648=CARTESIAN_POINT ( 'NONE',  ( -69.66297551618575312, -8.676591480033549075, 7.503902134509970345 ) ) ;
#21681=CARTESIAN_POINT ( 'NONE',  ( -67.26848159797359017, 2.000000000007965184, -1.381457631268952602 ) ) ;
#21792=CARTESIAN_POINT ( 'NONE',  ( -69.74732653341585831, -11.70592520059384256, -8.307376767094716286 ) ) ;
#21802=ORIENTED_EDGE ( 'NONE', *, *, #42215, .F. ) ;
#21864=EDGE_CURVE ( 'NONE', #37895, #46706, #49864, .T. ) ;
#21909=CYLINDRICAL_SURFACE ( 'NONE', #24112, 3.000000000000001332 ) ;
#21984=DIRECTION ( 'NONE',  ( 0.000000000000000000, -5.782411586589354681E-16, 1.000000000000000000 ) ) ;
#21987=EDGE_CURVE ( 'NONE', #4219, #26092, #52889, .T. ) ;
#22000=DIRECTION ( 'NONE',  ( 2.551063935260010306E-17, -5.102127870520020982E-16, 1.000000000000000000 ) ) ;
#22001=DIRECTION ( 'NONE',  ( 0.000000000000000000, 0.000000000000000000, 1.000000000000000000 ) ) ;
#22116=CARTESIAN_POINT ( 'NONE',  ( -65.59431828190201941, -5.464378949326942347E-14, 0.3363546178748699211 ) ) ;
#22151=( NAMED_UNIT ( * ) SI_UNIT ( $, .STERADIAN. ) SOLID_ANGLE_UNIT ( ) );
#22166=VECTOR ( 'NONE', #8212, 1000.000000000000000 ) ;
#22181=DIRECTION ( 'NONE',  ( -0.9983709377222390602, -0.05705673239519638146, 0.000000000000000000 ) ) ;
#22183=CARTESIAN_POINT ( 'NONE',  ( 0.000000000000000000, 2.000000000000000000, -2.125000000000000000 ) ) ;
#22234=CARTESIAN_POINT ( 'NONE',  ( -69.97056075661562602, 2.000000000000000000, -7.659292557883846442 ) ) ;
#22265=B_SPLINE_CURVE_WITH_KNOTS ( 'NONE', 3,
 ( #10533, #27856, #36636, #2259, #53948, #27263 ),
 .UNSPECIFIED., .F., .F.,
 ( 4, 2, 4 ),
 ( 0.000000000000000000, 0.0002007373455692541874, 0.0004014746911385083748 ),
 .UNSPECIFIED. ) ;
#22268=ORIENTED_EDGE ( 'NONE', *, *, #23221, .T. ) ;
#22287=DIRECTION ( 'NONE',  ( -0.1139275668495183524, 0.9934890585767659488, 4.694855797473114533E-16 ) ) ;
#22302=CARTESIAN_POINT ( 'NONE',  ( -70.03639332226748593, -0.2499667854710889425, -7.502502568033361463 ) ) ;
#22308=CARTESIAN_POINT ( 'NONE',  ( -66.62919651559374756, -8.730421935648388754, 1.346828299457899725 ) ) ;
#22349=VERTEX_POINT ( 'NONE', #52263 ) ;
#22376=CARTESIAN_POINT ( 'NONE',  ( 5.284380629179495692, -1.088761635349915657, -2.393572233197383881 ) ) ;
#22381=PRODUCT ( 'Curved Precision Cutting Blades', 'Curved Precision Cutting Blades', '', ( #3637 ) ) ;
#22401=DIRECTION ( 'NONE',  ( -0.000000000000000000, -1.000000000000000000, -0.000000000000000000 ) ) ;
#22412=AXIS2_PLACEMENT_3D ( 'NONE', #31571, #48029, #52835 ) ;
#22456=VERTEX_POINT ( 'NONE', #22706 ) ;
#22507=CARTESIAN_POINT ( 'NONE',  ( -69.53969258253385988, 1.152504438008073340, 7.491856536230704577 ) ) ;
#22528=CARTESIAN_POINT ( 'NONE',  ( -67.15417979359860112, 2.000000000000000444, 6.891331229949076764 ) ) ;
#22529=EDGE_CURVE ( 'NONE', #50240, #24558, #26495, .T. ) ;
#22581=CARTESIAN_POINT ( 'NONE',  ( -68.91359625414428081, -8.992215709865041262, 7.224037831218169003 ) ) ;
#22637=CARTESIAN_POINT ( 'NONE',  ( 5.907100548706921472, -1.017206782221826478, 1.544798379698097079 ) ) ;
#22650=CARTESIAN_POINT ( 'NONE',  ( -69.30403031588791407, -1.000000000000000666, -6.450409451741321298 ) ) ;
#22661=CARTESIAN_POINT ( 'NONE',  ( -67.57495167298797867, -9.577535775341699420, 4.288727116335238065 ) ) ;
#22664=EDGE_CURVE ( 'NONE', #43677, #5292, #41007, .T. ) ;
#22695=EDGE_LOOP ( 'NONE', ( #2602, #31879, #29090, #35297 ) ) ;
#22706=CARTESIAN_POINT ( 'NONE',  ( -70.10169143752739274, -0.9999999999999995559, 7.503902134509972122 ) ) ;
#22715=EDGE_CURVE ( 'NONE', #37895, #2677, #24797, .T. ) ;
#22733=ORIENTED_EDGE ( 'NONE', *, *, #48258, .T. ) ;
#22767=CARTESIAN_POINT ( 'NONE',  ( -67.27407007597652466, -11.42230648536675908, 4.403654818465663645 ) ) ;
#22809=CARTESIAN_POINT ( 'NONE',  ( -68.87050791938486327, -8.585715889274698753, -6.450409451741323075 ) ) ;
#22849=ADVANCED_FACE ( 'NONE', ( #48486 ), #17329, .T. ) ;
#22859=CARTESIAN_POINT ( 'NONE',  ( 5.515141197255969630, -1.062154408800312755, -2.500037664106760094 ) ) ;
#22925=CARTESIAN_POINT ( 'NONE',  ( -71.02048890987401819, -1.000000000000000000, 8.554889286408840832 ) ) ;
#22931=CARTESIAN_POINT ( 'NONE',  ( -68.61431715373868201, 1.786464687300608922, -7.472022508502793592 ) ) ;
#22952=EDGE_LOOP ( 'NONE', ( #25426, #7651, #26408, #35672 ) ) ;
#22958=CARTESIAN_POINT ( 'NONE',  ( -67.75126421527782838, -8.858758211978919661, -5.285932311690691776 ) ) ;
#22997=CARTESIAN_POINT ( 'NONE',  ( -68.93342745996714882, -0.9999999999999983347, -5.847034362371242189 ) ) ;
#23017=VERTEX_POINT ( 'NONE', #12903 ) ;
#23025=EDGE_CURVE ( 'NONE', #3658, #7825, #14624, .T. ) ;
#23040=EDGE_CURVE ( 'NONE', #43429, #3658, #34524, .T. ) ;
#23059=CARTESIAN_POINT ( 'NONE',  ( -67.99914138734528990, -9.626105528482602480, -5.294842188089768698 ) ) ;
#23063=CARTESIAN_POINT ( 'NONE',  ( -67.02267797893095747, -0.6010035547808885159, -0.3415480826665019953 ) ) ;
#23078=CARTESIAN_POINT ( 'NONE',  ( -66.07241458602462103, 2.000000000000034195, -4.498572511313228439 ) ) ;
#23142=CARTESIAN_POINT ( 'NONE',  ( -68.33899556999409697, -8.925864846846893741, -6.396357082918144421 ) ) ;
#23209=CARTESIAN_POINT ( 'NONE',  ( -69.02562660986798448, 0.1329415388989311775, 6.116987600435763284 ) ) ;
#23218=DIRECTION ( 'NONE',  ( 0.000000000000000000, 0.000000000000000000, -1.000000000000000000 ) ) ;
#23219=CARTESIAN_POINT ( 'NONE',  ( 0.3240706152708105470, -3.670543518250628079, -2.125000000000001332 ) ) ;
#23221=EDGE_CURVE ( 'NONE', #27104, #22456, #39248, .T. ) ;
#23225=CARTESIAN_POINT ( 'NONE',  ( -66.79270813916639327, 2.820013818116702216E-15, -3.456045872278595610 ) ) ;
#23226=ORIENTED_EDGE ( 'NONE', *, *, #54015, .F. ) ;
#23231=CARTESIAN_POINT ( 'NONE',  ( -67.79210531775262893, 2.000000000000010214, -7.454399636913916716 ) ) ;
#23332=CARTESIAN_POINT ( 'NONE',  ( -67.50702643244157741, 2.000000000000000000, -7.448289400635801805 ) ) ;
#23344=CARTESIAN_POINT ( 'NONE',  ( -69.22403449346161608, 1.440755222218420117, 7.485090880804399660 ) ) ;
#23350=CARTESIAN_POINT ( 'NONE',  ( -67.25378808574402001, -11.41998066427858483, 8.237893588737414063 ) ) ;
#23354=CARTESIAN_POINT ( 'NONE',  ( -66.10469148387817029, 7.155734338404329264E-14, -3.769581895381322934 ) ) ;
#23391=CARTESIAN_POINT ( 'NONE',  ( -69.40103061304014886, -8.646553156806547236, -7.175319846998990947 ) ) ;
#23425=CARTESIAN_POINT ( 'NONE',  ( -67.70181732770106464, -8.853663008591706074, -5.215119943113103673 ) ) ;
#23434=CARTESIAN_POINT ( 'NONE',  ( 5.273499422741863008, -1.089864486915345099, -2.388555951666875288 ) ) ;
#23477=PLANE ( 'NONE',  #55624 ) ;
#23559=CARTESIAN_POINT ( 'NONE',  ( 5.284044854955649129, -1.088655197871726710, 2.393421119419573806 ) ) ;
#23606=CARTESIAN_POINT ( 'NONE',  ( -67.60174820569504561, -9.580611907208711031, 4.357869429825873553 ) ) ;
#23610=CARTESIAN_POINT ( 'NONE',  ( -67.26227515700414017, 8.227372716571623961E-12, 4.538413701022403046 ) ) ;
#23663=CARTESIAN_POINT ( 'NONE',  ( -68.98024086217516526, -9.100687180210641714, 7.490399608206207205 ) ) ;
#23676=FACE_OUTER_BOUND ( 'NONE', #28051, .T. ) ;
#23724=ORIENTED_EDGE ( 'NONE', *, *, #49818, .T. ) ;
#23778=LINE ( 'NONE', #28318, #8624 ) ;
#23787=ORIENTED_EDGE ( 'NONE', *, *, #46101, .T. ) ;
#23828=LINE ( 'NONE', #11336, #31256 ) ;
#23879=CARTESIAN_POINT ( 'NONE',  ( -65.13378959736581919, -11.17687152541042295, -3.942473205280556670 ) ) ;
#23883=( BOUNDED_CURVE ( )  B_SPLINE_CURVE ( 3, ( #30298, #13269, #8422, #17809 ),
 .UNSPECIFIED., .F., .F. ) 
 B_SPLINE_CURVE_WITH_KNOTS ( ( 4, 4 ),
 ( 5.142782291042174769, 6.283185307179586232 ),
 .UNSPECIFIED. ) 
 CURVE ( )  GEOMETRIC_REPRESENTATION_ITEM ( )  RATIONAL_B_SPLINE_CURVE ( ( 1.000000000000000000, 0.8945281452387645604, 0.8945281452387645604, 1.000000000000000000 ) ) 
 REPRESENTATION_ITEM ( '' )  );
#23885=CARTESIAN_POINT ( 'NONE',  ( -68.21604434836798703, -0.6011028652887574486, 5.268187007956926848 ) ) ;
#23935=EDGE_CURVE ( 'NONE', #33308, #3658, #22265, .T. ) ;
#23960=CARTESIAN_POINT ( 'NONE',  ( -68.18492111507299569, 1.999999999999999556, 4.989023737097912914 ) ) ;
#24079=ORIENTED_EDGE ( 'NONE', *, *, #3224, .T. ) ;
#24083=CARTESIAN_POINT ( 'NONE',  ( -66.20463474764028433, -9.286562617286856280, -2.844731389947795286 ) ) ;
#24087=DIRECTION ( 'NONE',  ( -0.9983709377222390602, -0.05705673239519638146, 0.000000000000000000 ) ) ;
#24112=AXIS2_PLACEMENT_3D ( 'NONE', #7753, #25081, #42395 ) ;
#24155=CARTESIAN_POINT ( 'NONE',  ( -67.81626209598535127, 0.000000000000000000, 7.454917401049828918 ) ) ;
#24185=CARTESIAN_POINT ( 'NONE',  ( -67.48059261034040901, -0.6012577534369748511, -3.373741216793211262 ) ) ;
#24351=CARTESIAN_POINT ( 'NONE',  ( -65.98131617537119098, -9.260953737796825180, 1.428098984226591872 ) ) ;
#24355=CARTESIAN_POINT ( 'NONE',  ( -69.66297551618575312, -8.676591480033549075, 7.503902134509970345 ) ) ;
#24403=CARTESIAN_POINT ( 'NONE',  ( -67.27731269685068582, -9.409571107119717226, -7.454891809856700746 ) ) ;
#24412=EDGE_CURVE ( 'NONE', #45113, #36795, #37472, .T. ) ;
#24438=CARTESIAN_POINT ( 'NONE',  ( -68.96873366698683583, -11.61664068348967938, -7.382776467525443920 ) ) ;
#24457=ORIENTED_EDGE ( 'NONE', *, *, #28909, .F. ) ;
#24558=VERTEX_POINT ( 'NONE', #30515 ) ;
#24614=CARTESIAN_POINT ( 'NONE',  ( -67.99425556498525225, -9.491785959746023238, 8.455601507725486243 ) ) ;
#24698=FACE_OUTER_BOUND ( 'NONE', #27085, .T. ) ;
#24701=EDGE_LOOP ( 'NONE', ( #4942, #52322, #38753, #56010 ) ) ;
#24716=CARTESIAN_POINT ( 'NONE',  ( -68.30214028159727491, 2.081668171172168513E-14, 8.159882300546032141 ) ) ;
#24726=ORIENTED_EDGE ( 'NONE', *, *, #4274, .T. ) ;
#24759=B_SPLINE_CURVE_WITH_KNOTS ( 'NONE', 3,
 ( #55086, #46251, #54783, #7654, #11643, #42569, #54490, #33760, #3662, #38035, #50801, #38302, #32926, #46005, #55343, #55622, #34067, #50243, #7111, #24403 ),
 .UNSPECIFIED., .F., .F.,
 ( 4, 2, 2, 2, 2, 2, 2, 2, 2, 4 ),
 ( 6.071532165918829453E-18, 0.001980665692890086396, 0.003961331385780166719, 0.005941997078670247477, 0.006932329925115283085, 0.007922662771560321296, 0.009903328464450394247, 0.01188399415734046893, 0.01386465985023054015, 0.01584532554312061484 ),
 .UNSPECIFIED. ) ;
#24782=DIRECTION ( 'NONE',  ( -0.1139275668495183524, 0.9934890585767659488, 4.694855797473117491E-16 ) ) ;
#24797=CIRCLE ( 'NONE', #29345, 6.000000000000001776 ) ;
#24803=CARTESIAN_POINT ( 'NONE',  ( -69.06384020419240244, 0.1330099063031576490, -6.182688104192161305 ) ) ;
#24847=EDGE_CURVE ( 'NONE', #2618, #280, #31195, .T. ) ;
#24873=VECTOR ( 'NONE', #13044, 1000.000000000000114 ) ;
#24895=( BOUNDED_CURVE ( )  B_SPLINE_CURVE ( 3, ( #495, #27172, #39105, #39946 ),
 .UNSPECIFIED., .F., .F. ) 
 B_SPLINE_CURVE_WITH_KNOTS ( ( 4, 4 ),
 ( 5.898329122556059900, 6.283185307179586232 ),
 .UNSPECIFIED. ) 
 CURVE ( )  GEOMETRIC_REPRESENTATION_ITEM ( )  RATIONAL_B_SPLINE_CURVE ( ( 1.000000000000000000, 0.9876951826469673179, 0.9876951826469673179, 1.000000000000000000 ) ) 
 REPRESENTATION_ITEM ( '' )  );
#24911=DIRECTION ( 'NONE',  ( -0.1139275668495183386, 0.9934890585767658377, 4.694855797473113547E-16 ) ) ;
#24914=CARTESIAN_POINT ( 'NONE',  ( -66.74449147233332269, -11.36157748060019301, 7.448312483692313357 ) ) ;
#24918=CARTESIAN_POINT ( 'NONE',  ( -66.55855263966657276, -8.722205571141092406, -0.3415480826687185001 ) ) ;
#24934=FACE_BOUND ( 'NONE', #27758, .T. ) ;
#24935=CARTESIAN_POINT ( 'NONE',  ( -69.34476620134752523, -0.4004433531566040649, -7.487678583014045763 ) ) ;
#24946=VECTOR ( 'NONE', #40177, 1000.000000000000114 ) ;
#24951=DIRECTION ( 'NONE',  ( -8.881784197001252323E-16, 0.000000000000000000, -1.000000000000000000 ) ) ;
#24963=AXIS2_PLACEMENT_3D ( 'NONE', #9195, #44132, #5242 ) ;
#24973=ORIENTED_EDGE ( 'NONE', *, *, #28373, .F. ) ;
#25020=EDGE_CURVE ( 'NONE', #22456, #23017, #41840, .T. ) ;
#25023=DIRECTION ( 'NONE',  ( 0.000000000000000000, 0.000000000000000000, 1.000000000000000000 ) ) ;
#25081=DIRECTION ( 'NONE',  ( -0.1139275668495183524, 0.9934890585767659488, 4.694855797473114533E-16 ) ) ;
#25113=CARTESIAN_POINT ( 'NONE',  ( -66.97721288434047437, 1.999999999999990452, 6.550948917179798769 ) ) ;
#25195=CARTESIAN_POINT ( 'NONE',  ( -68.50231803695028532, -8.543494007632164156, -5.847034362371243965 ) ) ;
#25208=EDGE_LOOP ( 'NONE', ( #42520, #48147, #36668, #48921 ) ) ;
#25213=CARTESIAN_POINT ( 'NONE',  ( -66.84355256359847886, -8.754982504685631994, 2.715629364116394218 ) ) ;
#25224=EDGE_CURVE ( 'NONE', #43677, #45113, #47111, .T. ) ;
#25298=CARTESIAN_POINT ( 'NONE',  ( -67.26331940870433357, -11.42107366115092226, -8.215550190278584353 ) ) ;
#25300=CARTESIAN_POINT ( 'NONE',  ( -67.09849928827489407, 4.336808689942017736E-15, 6.231849021622052121 ) ) ;
#25311=VERTEX_POINT ( 'NONE', #35198 ) ;
#25325=( GEOMETRIC_REPRESENTATION_CONTEXT ( 3 ) GLOBAL_UNCERTAINTY_ASSIGNED_CONTEXT ( ( #2446 ) ) GLOBAL_UNIT_ASSIGNED_CONTEXT ( ( #16772, #8840, #22151 ) ) REPRESENTATION_CONTEXT ( 'NONE', 'WORKASPACE' ) );
#25356=CARTESIAN_POINT ( 'NONE',  ( -67.50810339439870233, 2.000000000000000000, 7.448312483692316022 ) ) ;
#25373=CARTESIAN_POINT ( 'NONE',  ( -68.62740991863962847, 1.999999999996196598, 5.667235587295348154 ) ) ;
#25416=LINE ( 'NONE', #4130, #53951 ) ;
#25426=ORIENTED_EDGE ( 'NONE', *, *, #9306, .T. ) ;
#25458=VERTEX_POINT ( 'NONE', #31759 ) ;
#25486=CARTESIAN_POINT ( 'NONE',  ( -68.75329340164451253, -8.572274407770869686, 6.394134653913044808 ) ) ;
#25521=CARTESIAN_POINT ( 'NONE',  ( 5.221828392167460642, 0.000000000000000000, -2.393421119419572918 ) ) ;
#25531=CARTESIAN_POINT ( 'NONE',  ( 5.912796793901484271, -6.204513306124835204, 2.260536671351836002 ) ) ;
#25563=DIRECTION ( 'NONE',  ( -0.1139275668495183524, 0.9934890585767659488, 4.694855797473114533E-16 ) ) ;
#25576=EDGE_CURVE ( 'NONE', #23017, #7084, #35620, .T. ) ;
#25623=STYLED_ITEM ( 'NONE', ( #5509 ), #2589 ) ;
#25636=CYLINDRICAL_SURFACE ( 'NONE', #8071, 3.000000000000001332 ) ;
#25641=CARTESIAN_POINT ( 'NONE',  ( -65.68698218762608576, 2.000000000000004441, 3.192571262220380124 ) ) ;
#25667=PRODUCT_DEFINITION ( 'UNKNOWN', '', #28076, #42725 ) ;
#25682=ORIENTED_EDGE ( 'NONE', *, *, #2315, .T. ) ;
#25687=CARTESIAN_POINT ( 'NONE',  ( -66.74342152241241877, -11.36145478494482042, -7.448289400635804469 ) ) ;
#25729=LINE ( 'NONE', #51295, #33713 ) ;
#25740=EDGE_CURVE ( 'NONE', #33706, #43208, #23883, .T. ) ;
#25772=FACE_OUTER_BOUND ( 'NONE', #14791, .T. ) ;
#25776=CARTESIAN_POINT ( 'NONE',  ( -67.14101802347384762, -8.387388012353506284, -2.442027903730112026 ) ) ;
#25777=ORIENTED_EDGE ( 'NONE', *, *, #9049, .F. ) ;
#25893=ORIENTED_EDGE ( 'NONE', *, *, #14445, .F. ) ;
#25906=VECTOR ( 'NONE', #11073, 1000.000000000000000 ) ;
#25951=CARTESIAN_POINT ( 'NONE',  ( -65.40680149495634055, 2.000000000000022204, -1.598589950280139727 ) ) ;
#25956=CARTESIAN_POINT ( 'NONE',  ( -67.79130742519731712, -0.6009124436974506711, 4.273291358077424107 ) ) ;
#25964=ORIENTED_EDGE ( 'NONE', *, *, #19561, .T. ) ;
#26092=VERTEX_POINT ( 'NONE', #44328 ) ;
#26101=CARTESIAN_POINT ( 'NONE',  ( -66.84292213857837339, -9.493652800274178460, 1.352000712394443305 ) ) ;
#26116=CARTESIAN_POINT ( 'NONE',  ( -67.13288019662928718, 3.903127820947823062E-15, -6.325180979151116212 ) ) ;
#26133=EDGE_CURVE ( 'NONE', #10708, #43608, #4455, .T. ) ;
#26134=CARTESIAN_POINT ( 'NONE',  ( -70.10219403106212610, -1.000000000000000666, -7.503912900124007912 ) ) ;
#26306=ORIENTED_EDGE ( 'NONE', *, *, #26133, .F. ) ;
#26326=CARTESIAN_POINT ( 'NONE',  ( -66.35525671198902842, -11.31694229433773735, 0.4315550088921851768 ) ) ;
#26347=CARTESIAN_POINT ( 'NONE',  ( -69.02283434725003985, -9.743503351218873121, 6.962762944060569836 ) ) ;
#26367=( BOUNDED_CURVE ( )  B_SPLINE_CURVE ( 3, ( #35492, #9948, #53645, #18169 ),
 .UNSPECIFIED., .F., .F. ) 
 B_SPLINE_CURVE_WITH_KNOTS ( ( 4, 4 ),
 ( 2.756736468966273446, 3.141592653589797113 ),
 .UNSPECIFIED. ) 
 CURVE ( )  GEOMETRIC_REPRESENTATION_ITEM ( )  RATIONAL_B_SPLINE_CURVE ( ( 1.000000000000000000, 0.9876951826469675400, 0.9876951826469675400, 1.000000000000000000 ) ) 
 REPRESENTATION_ITEM ( '' )  );
#26408=ORIENTED_EDGE ( 'NONE', *, *, #43551, .F. ) ;
#26463=LINE ( 'NONE', #38723, #51288 ) ;
#26495=CIRCLE ( 'NONE', #52794, 6.000000000000002665 ) ;
#26500=EDGE_CURVE ( 'NONE', #18417, #26092, #37678, .T. ) ;
#26543=AXIS2_PLACEMENT_3D ( 'NONE', #19832, #15553, #32883 ) ;
#26544=CARTESIAN_POINT ( 'NONE',  ( -68.70267651662487651, -8.968872329527044940, -6.959823595413025643 ) ) ;
#26558=CARTESIAN_POINT ( 'NONE',  ( 5.618093201498282063, -1.050357395465043364, -2.260480044901387764 ) ) ;
#26570=AXIS2_PLACEMENT_3D ( 'NONE', #5936, #1656, #48813 ) ;
#26605=CARTESIAN_POINT ( 'NONE',  ( 5.518825648885151480, -1.048584701394832619, -2.502082349829454877 ) ) ;
#26635=CARTESIAN_POINT ( 'NONE',  ( -67.24306867387670650, -9.539447468475627190, -3.347029521210262981 ) ) ;
#26638=EDGE_CURVE ( 'NONE', #11765, #280, #25729, .T. ) ;
#26672=ORIENTED_EDGE ( 'NONE', *, *, #25740, .T. ) ;
#26684=CARTESIAN_POINT ( 'NONE',  ( 0.4518049228021103203, -3.655895688227122076, 5.998622290806040702 ) ) ;
#26713=EDGE_LOOP ( 'NONE', ( #15609, #45351, #18188, #19173, #20345, #29847, #1379, #24457, #4694, #6675, #36048, #26672, #20666, #674, #24079, #50940 ) ) ;
#26715=FACE_OUTER_BOUND ( 'NONE', #47026, .T. ) ;
#26777=CARTESIAN_POINT ( 'NONE',  ( -66.06974441054278202, 2.000000000000016431, 4.495433075559859937 ) ) ;
#26803=CARTESIAN_POINT ( 'NONE',  ( -68.75329340164451253, -8.572274407770867910, 6.394134653913044808 ) ) ;
#26832=CARTESIAN_POINT ( 'NONE',  ( 5.618093201498282063, -1.050357395465043364, -2.260480044901387764 ) ) ;
#26842=CARTESIAN_POINT ( 'NONE',  ( -66.67098249761872353, -8.735215231846519046, 1.683582515887789066 ) ) ;
#26875=ORIENTED_EDGE ( 'NONE', *, *, #10192, .T. ) ;
#26916=ORIENTED_EDGE ( 'NONE', *, *, #30039, .F. ) ;
#26919=ADVANCED_FACE ( 'NONE', ( #2901, #50633, #38121 ), #55172, .T. ) ;
#26941=CARTESIAN_POINT ( 'NONE',  ( -66.78432981023388493, -9.486898575435347425, 0.6700356180039961362 ) ) ;
#26958=CARTESIAN_POINT ( 'NONE',  ( -66.57070431223807816, -9.328541353163785743, -6.245432549306846326 ) ) ;
#27039=CARTESIAN_POINT ( 'NONE',  ( -68.86860983449916773, 1.667510478463746004, 7.477472888882761737 ) ) ;
#27044=CARTESIAN_POINT ( 'NONE',  ( -67.40686789321162564, -11.43753496933752167, 4.727715060443837380 ) ) ;
#27071=CARTESIAN_POINT ( 'NONE',  ( 4.994031378522667985, 0.000000000000000000, 2.289010529401726668 ) ) ;
#27080=ADVANCED_FACE ( 'NONE', ( #51189 ), #21380, .T. ) ;
#27085=EDGE_LOOP ( 'NONE', ( #55900, #3365, #17301, #12035 ) ) ;
#27102=( NAMED_UNIT ( * ) SI_UNIT ( $, .STERADIAN. ) SOLID_ANGLE_UNIT ( ) );
#27104=VERTEX_POINT ( 'NONE', #29898 ) ;
#27111=CARTESIAN_POINT ( 'NONE',  ( -70.08024661842391367, -0.7499901437495212209, -7.503442492476274595 ) ) ;
#27117=CARTESIAN_POINT ( 'NONE',  ( -66.66796270868890417, -8.734742092342063557, -1.671631898859750720 ) ) ;
#27169=DIRECTION ( 'NONE',  ( 0.9932609354084158682, 0.1139014070068027212, 0.02142857142857160571 ) ) ;
#27172=CARTESIAN_POINT ( 'NONE',  ( 4.854282358214434545, 0.000000000000000000, 1.997863978257570228 ) ) ;
#27199=CARTESIAN_POINT ( 'NONE',  ( -66.84260698025838110, -9.493516685082097339, -1.367274824955978518 ) ) ;
#27247=CARTESIAN_POINT ( 'NONE',  ( -67.32595136268157887, -0.9999999999999978906, 0.5932824550257459473 ) ) ;
#27263=CARTESIAN_POINT ( 'NONE',  ( 5.618093201498282063, -1.050357395465043364, -2.260480044901387764 ) ) ;
#27289=AXIS2_PLACEMENT_3D ( 'NONE', #27839, #32379, #32900 ) ;
#27301=CARTESIAN_POINT ( 'NONE',  ( -67.71562085171136403, -9.593594598721105982, -4.676733487554993296 ) ) ;
#27359=DIRECTION ( 'NONE',  ( 1.776356839400250465E-15, 0.000000000000000000, -1.000000000000000000 ) ) ;
#27396=FACE_BOUND ( 'NONE', #15812, .T. ) ;
#27417=ORIENTED_EDGE ( 'NONE', *, *, #22529, .F. ) ;
#27424=ORIENTED_EDGE ( 'NONE', *, *, #48258, .F. ) ;
#27426=ORIENTED_EDGE ( 'NONE', *, *, #14097, .F. ) ;
#27429=CARTESIAN_POINT ( 'NONE',  ( 5.359786524431354948, 0.000000000000000000, 2.456654125669140765 ) ) ;
#27430=CARTESIAN_POINT ( 'NONE',  ( -67.02664427580020856, -11.39393312870849151, -7.454399636913917604 ) ) ;
#27444=CARTESIAN_POINT ( 'NONE',  ( -70.00279782826048347, 0.1332992376639058896, -7.501782499249456393 ) ) ;
#27461=CARTESIAN_POINT ( 'NONE',  ( -70.71258200891328727, -1.000000000000000000, 8.208045577613541255 ) ) ;
#27467=EDGE_CURVE ( 'NONE', #33250, #17419, #46391, .T. ) ;
#27493=FACE_OUTER_BOUND ( 'NONE', #5684, .T. ) ;
#27544=FACE_OUTER_BOUND ( 'NONE', #18326, .T. ) ;
#27591=CARTESIAN_POINT ( 'NONE',  ( -69.97756022945675625, 0.4191520680014513278, 7.501241569353455318 ) ) ;
#27598=CARTESIAN_POINT ( 'NONE',  ( -68.18449814332990400, -11.52670909917258690, -6.247493715003795245 ) ) ;
#27603=CARTESIAN_POINT ( 'NONE',  ( -66.73496964911797136, 1.799964814818122178E-11, 2.845885083211338262 ) ) ;
#27665=ORIENTED_EDGE ( 'NONE', *, *, #18047, .T. ) ;
#27672=CLOSED_SHELL ( 'NONE', ( #1795, #51154, #17072, #21565, #55733, #30221, #3165, #49444, #31876, #14752, #933, #27929, #33085, #55639, #22849, #38702, #39445, #19090, #4476, #3147, #9055, #46556, #26919, #27080, #35921, #19544, #15981, #55658, #10890, #37759, #34518, #4051, #6816, #17391, #37231, #45932, #42385 ) ) ;
#27739=CARTESIAN_POINT ( 'NONE',  ( 5.500940387028403933, 0.000000000000000000, 2.400892578144000922 ) ) ;
#27758=EDGE_LOOP ( 'NONE', ( #42638, #1024 ) ) ;
#27765=CARTESIAN_POINT ( 'NONE',  ( -71.01620612404938981, -1.000000000000001776, -8.550077602493738382 ) ) ;
#27771=CARTESIAN_POINT ( 'NONE',  ( -68.48236398700224470, 1.836504256775132404, -7.469194291234003025 ) ) ;
#27779=CARTESIAN_POINT ( 'NONE',  ( -70.12381838982661009, -8.729438269679169693, -8.047023921085742160 ) ) ;
#27821=VERTEX_POINT ( 'NONE', #34570 ) ;
#27839=CARTESIAN_POINT ( 'NONE',  ( -58.00000000000000711, 2.000000000000000000, 7.102951435054649637E-15 ) ) ;
#27856=CARTESIAN_POINT ( 'NONE',  ( 5.345667018682350502, -1.081588725305391074, -2.421850695157840239 ) ) ;
#27894=CARTESIAN_POINT ( 'NONE',  ( -66.74797292598515241, -11.36197671352631033, 2.764386752171343886 ) ) ;
#27897=( BOUNDED_SURFACE ( )  B_SPLINE_SURFACE ( 3, 2, ( 
 ( #49357, #10752, #48522 ),
 ( #44816, #9637, #6217 ),
 ( #6475, #41112, #2200 ),
 ( #26958, #44270, #31501 ),
 ( #1074, #53607, #22958 ),
 ( #10477, #40580, #36050 ),
 ( #49071, #32596, #29463 ),
 ( #11289, #15823, #3033 ),
 ( #16376, #24083, #20367 ),
 ( #49898, #46784, #16122 ),
 ( #42243, #7052, #3344 ),
 ( #55286, #7589, #2495 ),
 ( #20667, #45641, #24918 ),
 ( #6759, #37982, #19815 ),
 ( #41408, #45944, #50179 ),
 ( #33701, #24351, #37136 ),
 ( #15532, #11001, #28622 ),
 ( #41659, #51016, #25213 ),
 ( #54435, #29159, #41933 ),
 ( #12126, #7902, #2745 ),
 ( #54718, #20070, #33441 ),
 ( #32866, #42521, #50745 ),
 ( #37396, #55031, #19537 ),
 ( #36879, #11838, #33170 ),
 ( #50486, #11585, #28901 ),
 ( #54184, #37708, #46472 ),
 ( #15284, #46197, #7302 ),
 ( #24614, #28323, #42778 ) ),
 .UNSPECIFIED., .F., .F., .F. ) 
 B_SPLINE_SURFACE_WITH_KNOTS ( ( 4, 2, 2, 2, 2, 2, 2, 2, 2, 2, 2, 2, 2, 4 ),
 ( 3, 3 ),
 ( 0.005951394764495080564, 0.008223488340404870242, 0.009359535128359765949, 0.01049558191631465992, 0.01276767549222445133, 0.01390372228017934531, 0.01503976906813424101, 0.01617581585608913672, 0.01731186264404403069, 0.01958395621995382210, 0.02072000300790871608, 0.02185604979586361352, 0.02299209658381850749, 0.02412814337177340146 ),
 ( 0.000000000000000000, 1.000000000000000000 ),
 .UNSPECIFIED. ) 
 GEOMETRIC_REPRESENTATION_ITEM ( )  RATIONAL_B_SPLINE_SURFACE ( (
 ( 1.000000000000000000, 0.9218171296615468302, 1.000000000000000000),
 ( 1.000000000000000000, 0.9219582590430798197, 1.000000000000000000),
 ( 1.000000000000000000, 0.9217654209506799257, 1.000000000000000000),
 ( 1.000000000000000000, 0.9218193965221213038, 1.000000000000000000),
 ( 1.000000000000000000, 0.9217886515252998736, 1.000000000000000000),
 ( 1.000000000000000000, 0.9217705453229111390, 1.000000000000000000),
 ( 1.000000000000000000, 0.9217728555244316668, 1.000000000000000000),
 ( 1.000000000000000000, 0.9217839018303625176, 1.000000000000000000),
 ( 1.000000000000000000, 0.9217902773702886243, 1.000000000000000000),
 ( 1.000000000000000000, 0.9218159477367721122, 1.000000000000000000),
 ( 1.000000000000000000, 0.9218381644593317548, 1.000000000000000000),
 ( 1.000000000000000000, 0.9218170478688526570, 1.000000000000000000),
 ( 1.000000000000000000, 0.9218183721990944601, 1.000000000000000000),
 ( 1.000000000000000000, 0.9218243750419194971, 1.000000000000000000),
 ( 1.000000000000000000, 0.9218291361985332388, 1.000000000000000000),
 ( 1.000000000000000000, 0.9218339850781324119, 1.000000000000000000),
 ( 1.000000000000000000, 0.9218340914605103187, 1.000000000000000000),
 ( 1.000000000000000000, 0.9218311426340464187, 1.000000000000000000),
 ( 1.000000000000000000, 0.9218408506499762289, 1.000000000000000000),
 ( 1.000000000000000000, 0.9218298856244220296, 1.000000000000000000),
 ( 1.000000000000000000, 0.9218235216675588761, 1.000000000000000000),
 ( 1.000000000000000000, 0.9218049054827647248, 1.000000000000000000),
 ( 1.000000000000000000, 0.9217926302233848679, 1.000000000000000000),
 ( 1.000000000000000000, 0.9217749384510963706, 1.000000000000000000),
 ( 1.000000000000000000, 0.9217695517188546628, 1.000000000000000000),
 ( 1.000000000000000000, 0.9217886187906820794, 1.000000000000000000),
 ( 1.000000000000000000, 0.9218984684751962977, 1.000000000000000000),
 ( 1.000000000000000000, 0.9217608302862904113, 1.000000000000000000) ) ) 
 REPRESENTATION_ITEM ( '' )  SURFACE ( )  );
#27899=CARTESIAN_POINT ( 'NONE',  ( -65.67246414475930294, 5.724587470723463412E-14, -1.520040349668396962 ) ) ;
#27914=CARTESIAN_POINT ( 'NONE',  ( -65.57067994458799376, 1.999999999999980904, 2.608662443145409071 ) ) ;
#27929=ADVANCED_FACE ( 'NONE', ( #8183 ), #39699, .F. ) ;
#27957=CARTESIAN_POINT ( 'NONE',  ( 5.907100043276122037, -1.017206840181698935, -1.544800305917336303 ) ) ;
#27967=CARTESIAN_POINT ( 'NONE',  ( -70.07530963300145288, 1.999999999999999112, -7.815307374640574345 ) ) ;
#27980=CARTESIAN_POINT ( 'NONE',  ( 5.850167639498142336, 0.0001172167714158106350, -1.544991171441945532 ) ) ;
#28051=EDGE_LOOP ( 'NONE', ( #5094, #27665, #16893, #36557 ) ) ;
#28076=PRODUCT_DEFINITION_FORMATION_WITH_SPECIFIED_SOURCE ( 'ANY', '', #22381, .NOT_KNOWN. ) ;
#28148=CARTESIAN_POINT ( 'NONE',  ( -68.37432498243255452, -0.6009960021135252184, -5.589544126886995201 ) ) ;
#28216=CARTESIAN_POINT ( 'NONE',  ( -70.56555449637278343, -1.000000000000001332, -8.047023921085740383 ) ) ;
#28281=DIRECTION ( 'NONE',  ( -0.000000000000000000, -1.000000000000000000, -0.000000000000000000 ) ) ;
#28293=DIRECTION ( 'NONE',  ( -0.1139275668495183524, 0.9934890585767659488, 4.694855797473114533E-16 ) ) ;
#28318=CARTESIAN_POINT ( 'NONE',  ( -57.29829478218162109, -10.27834239552269580, -2.999999999999996891 ) ) ;
#28323=CARTESIAN_POINT ( 'NONE',  ( -68.64911863573352946, -9.566881861030363865, 7.932749270814273501 ) ) ;
#28351=VECTOR ( 'NONE', #32242, 1000.000000000000114 ) ;
#28373=EDGE_CURVE ( 'NONE', #26092, #4219, #36566, .T. ) ;
#28406=AXIS2_PLACEMENT_3D ( 'NONE', #15118, #40927, #44622 ) ;
#28423=CARTESIAN_POINT ( 'NONE',  ( -65.91414241012756747, -5.204170427930421283E-15, -3.032880804699297439 ) ) ;
#28424=ORIENTED_EDGE ( 'NONE', *, *, #22664, .F. ) ;
#28446=ORIENTED_EDGE ( 'NONE', *, *, #1413, .F. ) ;
#28501=DIRECTION ( 'NONE',  ( -0.000000000000000000, -1.000000000000000000, -0.000000000000000000 ) ) ;
#28622=CARTESIAN_POINT ( 'NONE',  ( -66.67378107351682104, -8.735535983216148992, 1.704803601108932920 ) ) ;
#28627=CARTESIAN_POINT ( 'NONE',  ( -69.43545830293986398, -9.790829293527439248, 7.501778215771295777 ) ) ;
#28671=DIRECTION ( 'NONE',  ( -0.9932609354084158682, -0.1139014070068027212, -0.02142857142857160571 ) ) ;
#28725=DIRECTION ( 'NONE',  ( 0.000000000000000000, 1.000000000000000000, 0.000000000000000000 ) ) ;
#28728=CARTESIAN_POINT ( 'NONE',  ( -67.26768186997090027, -3.935216494285589413E-12, -4.549856479222408545 ) ) ;
#28739=DIRECTION ( 'NONE',  ( -0.000000000000000000, -1.000000000000000000, -0.000000000000000000 ) ) ;
#28800=CARTESIAN_POINT ( 'NONE',  ( -67.27906308014451042, 1.999999999999999556, 2.024546322512588148 ) ) ;
#28801=LINE ( 'NONE', #41826, #38719 ) ;
#28882=CARTESIAN_POINT ( 'NONE',  ( -67.38882915104511540, -9.422359167723826090, 6.206396125462540603 ) ) ;
#28901=CARTESIAN_POINT ( 'NONE',  ( -68.39955523751335420, -8.932958699260208135, 6.466593069173195651 ) ) ;
#28909=EDGE_CURVE ( 'NONE', #8945, #16356, #49295, .T. ) ;
#28932=ORIENTED_EDGE ( 'NONE', *, *, #28909, .T. ) ;
#29031=FACE_OUTER_BOUND ( 'NONE', #6235, .T. ) ;
#29058=CARTESIAN_POINT ( 'NONE',  ( -70.75814845257580998, 2.000000000000000000, 8.563005977519216216 ) ) ;
#29085=ORIENTED_EDGE ( 'NONE', *, *, #40217, .T. ) ;
#29090=ORIENTED_EDGE ( 'NONE', *, *, #14445, .T. ) ;
#29159=CARTESIAN_POINT ( 'NONE',  ( -66.37927290664002555, -9.306589109140311677, 3.533109812937361927 ) ) ;
#29162=EDGE_CURVE ( 'NONE', #280, #2618, #44755, .T. ) ;
#29329=DIRECTION ( 'NONE',  ( -2.683102249366423030E-17, 4.694855797473116505E-16, -1.000000000000000000 ) ) ;
#29345=AXIS2_PLACEMENT_3D ( 'NONE', #35177, #51625, #17256 ) ;
#29346=FACE_OUTER_BOUND ( 'NONE', #22952, .T. ) ;
#29350=CARTESIAN_POINT ( 'NONE',  ( -67.57167971728060252, 1.999999999999992673, -7.559434449104583287 ) ) ;
#29399=DIRECTION ( 'NONE',  ( 0.000000000000000000, 0.000000000000000000, -1.000000000000000000 ) ) ;
#29410=DIRECTION ( 'NONE',  ( -0.1139275668495183524, 0.9934890585767659488, 4.694855797473114533E-16 ) ) ;
#29412=CARTESIAN_POINT ( 'NONE',  ( 5.523400311179926803, 0.000000000000000000, -2.340279943148938724 ) ) ;
#29451=CARTESIAN_POINT ( 'NONE',  ( 4.530337070483293260, 0.000000000000000000, 2.076476591771610369 ) ) ;
#29458=CARTESIAN_POINT ( 'NONE',  ( -65.54186449640286583, -11.22366718957837683, 5.111569279459596160 ) ) ;
#29463=CARTESIAN_POINT ( 'NONE',  ( -67.34857948837910158, -8.812463414701275255, -4.340774506263340271 ) ) ;
#29466=CARTESIAN_POINT ( 'NONE',  ( -68.63714112026566738, -10.92288908917430312, -7.487543234984625151 ) ) ;
#29480=CARTESIAN_POINT ( 'NONE',  ( -70.57579075201010710, -8.781267840485488918, 8.554889286408839055 ) ) ;
#29551=AXIS2_PLACEMENT_3D ( 'NONE', #39536, #30157, #17360 ) ;
#29663=CARTESIAN_POINT ( 'NONE',  ( -68.27148781930287669, 0.1328899438206843642, -4.676733487538881739 ) ) ;
#29708=DIRECTION ( 'NONE',  ( -0.000000000000000000, -1.000000000000000000, -0.000000000000000000 ) ) ;
#29729=( BOUNDED_CURVE ( )  B_SPLINE_CURVE ( 3, ( #33512, #54506, #46020, #3115 ),
 .UNSPECIFIED., .F., .F. ) 
 B_SPLINE_CURVE_WITH_KNOTS ( ( 4, 4 ),
 ( 1.527237336719642125, 1.527316689203489508 ),
 .UNSPECIFIED. ) 
 CURVE ( )  GEOMETRIC_REPRESENTATION_ITEM ( )  RATIONAL_B_SPLINE_CURVE ( ( 1.000000000000000000, 0.9999999994752652999, 0.9999999994752652999, 1.000000000000000000 ) ) 
 REPRESENTATION_ITEM ( '' )  );
#29735=DIRECTION ( 'NONE',  ( -0.9983709377222390602, -0.05705673239519638146, 0.000000000000000000 ) ) ;
#29740=CARTESIAN_POINT ( 'NONE',  ( -68.90235146048875947, -9.595921133603816600, 8.251517284182451561 ) ) ;
#29746=EDGE_CURVE ( 'NONE', #33250, #23017, #21433, .T. ) ;
#29775=CARTESIAN_POINT ( 'NONE',  ( -68.07298578174265913, -11.51392150788243818, -6.094799798532272384 ) ) ;
#29792=CARTESIAN_POINT ( 'NONE',  ( -58.00000000000000711, 2.000000000000000000, -2.999999999999994227 ) ) ;
#29795=CARTESIAN_POINT ( 'NONE',  ( 4.966775449259090536, -1.125037814383458512, -2.247047898273223598 ) ) ;
#29836=CARTESIAN_POINT ( 'NONE',  ( -69.59783862807636012, -0.6008070088998225255, -7.493102809087827332 ) ) ;
#29845=SURFACE_SIDE_STYLE ('',( #17316 ) ) ;
#29846=CARTESIAN_POINT ( 'NONE',  ( -68.97544431584221059, -1.373506146286891395E-11, 7.657917462049396384 ) ) ;
#29847=ORIENTED_EDGE ( 'NONE', *, *, #34373, .T. ) ;
#29898=CARTESIAN_POINT ( 'NONE',  ( -70.00259797851279586, 0.1329035588801656675, 7.501778215771297553 ) ) ;
#29908=CARTESIAN_POINT ( 'NONE',  ( 5.577510371788088506, -6.223674869166637258, 2.393421119419572474 ) ) ;
#29912=VERTEX_POINT ( 'NONE', #4917 ) ;
#29917=CARTESIAN_POINT ( 'NONE',  ( -68.17482077307661825, 1.999999999996754596, 4.727715060444682926 ) ) ;
#29921=CARTESIAN_POINT ( 'NONE',  ( -69.49476718086417293, -0.5994838070687775744, 7.360527835276493569 ) ) ;
#29931=CARTESIAN_POINT ( 'NONE',  ( -69.48114687386605226, -8.789460189087408892, -7.500305896622815105 ) ) ;
#29995=B_SPLINE_CURVE_WITH_KNOTS ( 'NONE', 3,
 ( #2904, #5884, #33583, #20234, #37870, #55174, #23209, #11728, #36007, #16264, #36261, #54892, #16004, #46347, #50893, #31722, #11994, #53316, #49025, #53562, #10125, #27444 ),
 .UNSPECIFIED., .F., .F.,
 ( 4, 2, 2, 2, 2, 2, 2, 2, 2, 2, 4 ),
 ( -5.999998108584347237E-08, 0.0005071597037827979635, 0.001014379407546681881, 0.002028818815074472700, 0.003043258222602263953, 0.004057697630130054772, 0.006086576445185653758, 0.008115455260241252744, 0.01014433407529685346, 0.01217321289035245419, 0.01623097052046365216 ),
 .UNSPECIFIED. ) ;
#30021=ORIENTED_EDGE ( 'NONE', *, *, #23935, .T. ) ;
#30027=EDGE_CURVE ( 'NONE', #54422, #16523, #23828, .T. ) ;
#30039=EDGE_CURVE ( 'NONE', #12427, #4219, #50786, .T. ) ;
#30049=SHAPE_DEFINITION_REPRESENTATION ( #53650, #53575 ) ;
#30081=CARTESIAN_POINT ( 'NONE',  ( -65.59269431991148736, -5.464378949326944241E-14, -0.6466721865751011711 ) ) ;
#30146=ORIENTED_EDGE ( 'NONE', *, *, #21864, .F. ) ;
#30157=DIRECTION ( 'NONE',  ( 0.000000000000000000, 1.000000000000000000, 0.000000000000000000 ) ) ;
#30190=CARTESIAN_POINT ( 'NONE',  ( -69.24581943945996443, 0.1330540280733476244, -6.471852447751588855 ) ) ;
#30197=EDGE_CURVE ( 'NONE', #24558, #10708, #21558, .T. ) ;
#30214=DIRECTION ( 'NONE',  ( 0.000000000000000000, 1.000000000000000000, 0.000000000000000000 ) ) ;
#30221=ADVANCED_FACE ( 'NONE', ( #7841 ), #42467, .F. ) ;
#30241=AXIS2_PLACEMENT_3D ( 'NONE', #47234, #30214, #3253 ) ;
#30298=CARTESIAN_POINT ( 'NONE',  ( 4.994031378522669762, 0.000000000000000000, -2.289010529401725780 ) ) ;
#30433=EDGE_LOOP ( 'NONE', ( #9335, #54358, #31534, #55351, #28932, #5477, #32732, #47301 ) ) ;
#30444=EDGE_CURVE ( 'NONE', #4538, #13662, #25416, .T. ) ;
#30446=CIRCLE ( 'NONE', #29551, 2.125000000000000000 ) ;
#30494=CARTESIAN_POINT ( 'NONE',  ( -67.20861331203366262, 1.999999999987024379, -0.6963329337696058108 ) ) ;
#30513=CARTESIAN_POINT ( 'NONE',  ( -69.11692417668358246, -9.015782624321049710, -7.493102809087829108 ) ) ;
#30515=CARTESIAN_POINT ( 'NONE',  ( 0.2239497891030726440, -1.668917571073584849, -5.998622290806042479 ) ) ;
#30545=CIRCLE ( 'NONE', #19621, 3.000000000000001332 ) ;
#30565=DIRECTION ( 'NONE',  ( 0.000000000000000000, 0.000000000000000000, -1.000000000000000000 ) ) ;
#30580=EDGE_CURVE ( 'NONE', #43208, #42953, #37669, .T. ) ;
#30646=CARTESIAN_POINT ( 'NONE',  ( -68.58058681874440765, -9.692212885547005996, -6.443496511055998077 ) ) ;
#30661=CARTESIAN_POINT ( 'NONE',  ( -65.97216590917611256, 4.336808689942016158E-15, -3.251835480715624893 ) ) ;
#30665=CARTESIAN_POINT ( 'NONE',  ( 5.359786524431358501, 0.000000000000000000, -2.456654125669140321 ) ) ;
#30715=( BOUNDED_CURVE ( )  B_SPLINE_CURVE ( 3, ( #13977, #39561, #4617, #653 ),
 .UNSPECIFIED., .F., .F. ) 
 B_SPLINE_CURVE_WITH_KNOTS ( ( 4, 4 ),
 ( 3.141592653589797113, 3.526448838213318115 ),
 .UNSPECIFIED. ) 
 CURVE ( )  GEOMETRIC_REPRESENTATION_ITEM ( )  RATIONAL_B_SPLINE_CURVE ( ( 1.000000000000000000, 0.9876951826469675400, 0.9876951826469675400, 1.000000000000000000 ) ) 
 REPRESENTATION_ITEM ( '' )  );
#30732=AXIS2_PLACEMENT_3D ( 'NONE', #21090, #47212, #17392 ) ;
#30745=CARTESIAN_POINT ( 'NONE',  ( -68.99096209019747050, 1.598546839610802461, 7.480095325092517733 ) ) ;
#30816=CARTESIAN_POINT ( 'NONE',  ( -68.71918076694248612, -8.969740930377138710, 6.949370683160943862 ) ) ;
#30824=EDGE_LOOP ( 'NONE', ( #53191, #43222, #29085, #11244, #30021, #42061, #50175, #5486, #18396, #18830, #51454, #27426, #14104, #22733, #42355, #31215 ) ) ;
#30852=EDGE_LOOP ( 'NONE', ( #40991, #47965, #3596, #25682, #27417, #6348, #17227, #17948 ) ) ;
#30868=CARTESIAN_POINT ( 'NONE',  ( 5.283022392374841836, -1.075897820612792044, -2.393286648641791636 ) ) ;
#30889=CARTESIAN_POINT ( 'NONE',  ( -69.43561177275644525, -9.791245164465275153, -7.501782499249458169 ) ) ;
#30908=CARTESIAN_POINT ( 'NONE',  ( -67.45300034126424293, 4.561518438557346199E-46, -6.901381173728422525 ) ) ;
#30934=CARTESIAN_POINT ( 'NONE',  ( -69.66297551618575312, -8.676591480033549075, 7.503902134509970345 ) ) ;
#31022=EDGE_CURVE ( 'NONE', #33706, #48284, #26463, .T. ) ;
#31047=CARTESIAN_POINT ( 'NONE',  ( -69.53087401356451380, -8.661442845389931477, -7.341494710781373279 ) ) ;
#31148=CARTESIAN_POINT ( 'NONE',  ( 5.617234462649089544, -1.043562741351909740, -2.260263880414688842 ) ) ;
#31195=CIRCLE ( 'NONE', #15745, 3.000000000000001332 ) ;
#31215=ORIENTED_EDGE ( 'NONE', *, *, #8809, .T. ) ;
#31256=VECTOR ( 'NONE', #28671, 1000.000000000000114 ) ;
#31321=CARTESIAN_POINT ( 'NONE',  ( -65.33883713333176502, 2.000000000000018208, 0.6542134465202600335 ) ) ;
#31399=ORIENTED_EDGE ( 'NONE', *, *, #25576, .F. ) ;
#31419=VECTOR ( 'NONE', #55180, 1000.000000000000000 ) ;
#31428=LINE ( 'NONE', #55621, #21193 ) ;
#31472=CARTESIAN_POINT ( 'NONE',  ( -70.38892378062969613, -1.000000000000149436, 7.852029984319922384 ) ) ;
#31486=CARTESIAN_POINT ( 'NONE',  ( -68.64163227075424345, -9.699815782473507397, 6.404540763468498099 ) ) ;
#31501=CARTESIAN_POINT ( 'NONE',  ( -67.90139828824541723, -8.876202928981230755, -5.589544126885695796 ) ) ;
#31505=EDGE_LOOP ( 'NONE', ( #46001, #26875, #49749, #41532, #47282 ) ) ;
#31509=B_SPLINE_CURVE_WITH_KNOTS ( 'NONE', 3,
 ( #55514, #38195, #29412, #50966 ),
 .UNSPECIFIED., .F., .F.,
 ( 4, 4 ),
 ( 0.000000000000000000, 1.000000000000000000 ),
 .UNSPECIFIED. ) ;
#31534=ORIENTED_EDGE ( 'NONE', *, *, #46101, .F. ) ;
#31548=DIRECTION ( 'NONE',  ( -0.9997703818010067467, 0.000000000000000000, 0.02142857142857158143 ) ) ;
#31554=EDGE_LOOP ( 'NONE', ( #45860, #41782, #10755, #25893 ) ) ;
#31561=DIRECTION ( 'NONE',  ( 0.000000000000000000, -5.782411586589354681E-16, 1.000000000000000000 ) ) ;
#31571=CARTESIAN_POINT ( 'NONE',  ( 0.3240706152708106025, -3.670543518250628967, -1.335466778558061241E-15 ) ) ;
#31593=CARTESIAN_POINT ( 'NONE',  ( -68.02159960128747684, -9.628770505094481180, 5.304050906517969288 ) ) ;
#31635=B_SPLINE_CURVE_WITH_KNOTS ( 'NONE', 1,
 ( #28627, #24355 ),
 .UNSPECIFIED., .F., .F.,
 ( 2, 2 ),
 ( 0.001874228446202059594, 0.003011459512596941206 ),
 .UNSPECIFIED. ) ;
#31667=CARTESIAN_POINT ( 'NONE',  ( -68.17944635737889314, -8.907771540513445885, 6.097755213354407289 ) ) ;
#31715=CARTESIAN_POINT ( 'NONE',  ( -68.13647802434893208, -11.18517250923651574, -7.477522605581023996 ) ) ;
#31722=CARTESIAN_POINT ( 'NONE',  ( -67.33383789142597209, 0.1329135175168457139, -0.6948190221874496197 ) ) ;
#31734=CARTESIAN_POINT ( 'NONE',  ( -69.12566734621377407, -1.678475092257100935E-13, 7.875383342262419539 ) ) ;
#31759=CARTESIAN_POINT ( 'NONE',  ( -67.81506811452879901, 0.000000000000000000, -7.454891809856698970 ) ) ;
#31760=ORIENTED_EDGE ( 'NONE', *, *, #6156, .F. ) ;
#31790=LINE ( 'NONE', #10202, #45193 ) ;
#31849=CARTESIAN_POINT ( 'NONE',  ( -67.67563256367881763, -11.46835534393823686, -5.350280945795687693 ) ) ;
#31853=CARTESIAN_POINT ( 'NONE',  ( -65.91359709181411120, -3.035766082959412415E-14, 3.032081494009100986 ) ) ;
#31876=ADVANCED_FACE ( 'NONE', ( #35107 ), #13230, .T. ) ;
#31879=ORIENTED_EDGE ( 'NONE', *, *, #22664, .T. ) ;
#31903=AXIS2_PLACEMENT_3D ( 'NONE', #11159, #24782, #29329 ) ;
#31905=CARTESIAN_POINT ( 'NONE',  ( -1.246832498358330099E-15, 0.000000000000000000, 0.000000000000000000 ) ) ;
#32005=CARTESIAN_POINT ( 'NONE',  ( -67.98273966911209243, -0.9999999999999983347, -3.909888324369924284 ) ) ;
#32006=ORIENTED_EDGE ( 'NONE', *, *, #55504, .T. ) ;
#32011=CARTESIAN_POINT ( 'NONE',  ( -70.00279782826048347, 0.1332992376639058896, -7.501782499249456393 ) ) ;
#32075=AXIS2_PLACEMENT_3D ( 'NONE', #45906, #28293, #7023 ) ;
#32141=CARTESIAN_POINT ( 'NONE',  ( -66.44890184452549420, -11.32768097537891272, 0.7018102913113006824 ) ) ;
#32145=CARTESIAN_POINT ( 'NONE',  ( -66.91114292034374955, -1.627825983345676869E-11, 3.533109812942180739 ) ) ;
#32222=CARTESIAN_POINT ( 'NONE',  ( -68.44026216309750055, -1.000000000000000000, 5.059064008999124340 ) ) ;
#32239=CARTESIAN_POINT ( 'NONE',  ( 6.001673287911728494, 0.0004827855869357527193, -0.7726386493456292026 ) ) ;
#32242=DIRECTION ( 'NONE',  ( -0.05705673239519650636, 0.9983709377222390602, 2.351258244848514932E-16 ) ) ;
#32379=DIRECTION ( 'NONE',  ( 0.000000000000000000, 1.000000000000000000, 0.000000000000000000 ) ) ;
#32416=CARTESIAN_POINT ( 'NONE',  ( 5.385059872733033437, 0.000000000000000000, 0.6896135826588394302 ) ) ;
#32435=CARTESIAN_POINT ( 'NONE',  ( -64.65687102648206519, -11.12218126798172690, -1.598589950288901385 ) ) ;
#32439=CARTESIAN_POINT ( 'NONE',  ( -65.59416307815027380, 4.336808689942017736E-15, 0.3806443636350875237 ) ) ;
#32481=EDGE_CURVE ( 'NONE', #7084, #46706, #46584, .T. ) ;
#32512=VERTEX_POINT ( 'NONE', #3443 ) ;
#32574=CARTESIAN_POINT ( 'NONE',  ( -69.54161822237450963, 1.150459406892988756, -7.491897809418650134 ) ) ;
#32596=CARTESIAN_POINT ( 'NONE',  ( -66.73349045206065000, -9.347208724145792402, -4.549856479217463168 ) ) ;
#32636=B_SPLINE_CURVE_WITH_KNOTS ( 'NONE', 3,
 ( #36225, #53527, #36485, #53802, #33365, #50926, #20579, #19991, #42146, #33616, #37609, #50393, #33071, #6670 ),
 .UNSPECIFIED., .F., .F.,
 ( 4, 2, 2, 2, 2, 2, 4 ),
 ( 1.387778780781443673E-17, 0.0008437472854879791203, 0.001265620928231961416, 0.001687494570975943495, 0.002109368213719925791, 0.002531241856463908087, 0.003374989141951898700 ),
 .UNSPECIFIED. ) ;
#32679=CARTESIAN_POINT ( 'NONE',  ( -65.54473273541158562, -11.22399610260319314, 5.092367036313483197 ) ) ;
#32683=CARTESIAN_POINT ( 'NONE',  ( -67.03785620394307898, -0.6009241746136663176, 0.6802539881083679019 ) ) ;
#32717=VERTEX_POINT ( 'NONE', #23559 ) ;
#32732=ORIENTED_EDGE ( 'NONE', *, *, #22715, .F. ) ;
#32733=EDGE_CURVE ( 'NONE', #47190, #17834, #26367, .T. ) ;
#32812=B_SPLINE_CURVE_WITH_KNOTS ( 'NONE', 3,
 ( #43663, #43953, #13025, #26347, #51904, #31486, #48797, #13579, #44252, #4506, #22661, #47946, #9894, #26101, #26941, #4246, #27199, #21559, #26635, #38874, #30646, #30889 ),
 .UNSPECIFIED., .F., .F.,
 ( 4, 2, 2, 2, 2, 2, 2, 2, 2, 2, 4 ),
 ( -5.999998108584347237E-08, 0.0005071597037828261528, 0.001014379407546738259, 0.002028818815074536885, 0.003043258222602335077, 0.004057697630130134570, 0.006086576445185719678, 0.008115455260241304786, 0.01014433407529688989, 0.01217321289035247674, 0.01623097052046364869 ),
 .UNSPECIFIED. ) ;
#32866=CARTESIAN_POINT ( 'NONE',  ( -66.39500965126839560, -9.308393707792198768, 5.887047890946016437 ) ) ;
#32883=DIRECTION ( 'NONE',  ( -2.551063935260010306E-17, 4.081702296416016490E-16, -1.000000000000000000 ) ) ;
#32898=DIRECTION ( 'NONE',  ( 0.000000000000000000, 1.000000000000000000, 0.000000000000000000 ) ) ;
#32900=DIRECTION ( 'NONE',  ( 0.000000000000000000, 0.000000000000000000, 1.000000000000000000 ) ) ;
#32911=CARTESIAN_POINT ( 'NONE',  ( 0.3240706152708105470, -3.670543518250628079, -2.125000000000001332 ) ) ;
#32926=CARTESIAN_POINT ( 'NONE',  ( -65.11529574170205592, -9.161643534026593372, -1.301894315629610555 ) ) ;
#32970=CARTESIAN_POINT ( 'NONE',  ( -67.30955648132578517, -0.6009093778043306244, 2.715629364103489873 ) ) ;
#33015=DIRECTION ( 'NONE',  ( -0.02128905125521658726, -0.002441305003917799629, -0.9997703818010066357 ) ) ;
#33058=CARTESIAN_POINT ( 'NONE',  ( 5.551076415483179538, -1.058033566259081848, 2.420903282225134401 ) ) ;
#33071=CARTESIAN_POINT ( 'NONE',  ( -69.37797197704281871, -10.07236156554400353, 7.501241569353456207 ) ) ;
#33085=ADVANCED_FACE ( 'NONE', ( #44501 ), #35724, .F. ) ;
#33170=CARTESIAN_POINT ( 'NONE',  ( -68.22449927491872756, -8.912924279275781458, 6.175865180868210125 ) ) ;
#33184=AXIS2_PLACEMENT_3D ( 'NONE', #52810, #13916, #31548 ) ;
#33204=ORIENTED_EDGE ( 'NONE', *, *, #38278, .T. ) ;
#33250=VERTEX_POINT ( 'NONE', #54924 ) ;
#33274=CARTESIAN_POINT ( 'NONE',  ( -68.76879270600605309, -7.224796368693941748E-12, 7.369622379056993466 ) ) ;
#33282=CARTESIAN_POINT ( 'NONE',  ( 0.1285714285714296967, 0.000000000000000000, 5.998622290806041590 ) ) ;
#33308=VERTEX_POINT ( 'NONE', #51513 ) ;
#33315=DIRECTION ( 'NONE',  ( 0.000000000000000000, 1.000000000000000000, 0.000000000000000000 ) ) ;
#33342=CARTESIAN_POINT ( 'NONE',  ( -70.11839600776268355, -1.000000000000000222, -7.555920072494595630 ) ) ;
#33363=CARTESIAN_POINT ( 'NONE',  ( -69.66347483736342383, -8.676648739292067702, -7.503912900124009688 ) ) ;
#33365=CARTESIAN_POINT ( 'NONE',  ( -67.86660508942482295, -11.27593752063030053, 7.471997583267847354 ) ) ;
#33433=CARTESIAN_POINT ( 'NONE',  ( -68.13739796841800000, -7.564004218980900450E-15, 7.461800464507161834 ) ) ;
#33441=CARTESIAN_POINT ( 'NONE',  ( -67.46750306152793542, -8.826476960856009413, 4.644600239863266644 ) ) ;
#33446=ORIENTED_EDGE ( 'NONE', *, *, #26638, .F. ) ;
#33512=CARTESIAN_POINT ( 'NONE',  ( 5.282355347525632183, -1.069580340602398705, -2.393146392891059460 ) ) ;
#33525=CARTESIAN_POINT ( 'NONE',  ( -69.38651902536496152, -9.785563849073980691, -7.442420802397360369 ) ) ;
#33583=CARTESIAN_POINT ( 'NONE',  ( -69.79011221730237935, 0.1328921168376125672, 7.235198260161163297 ) ) ;
#33600=CARTESIAN_POINT ( 'NONE',  ( -69.14117849623558243, 2.000000000007579271, 6.564485215139889362 ) ) ;
#33616=CARTESIAN_POINT ( 'NONE',  ( -68.85940620956198188, -10.75105392561086859, 7.491856536230701025 ) ) ;
#33681=CARTESIAN_POINT ( 'NONE',  ( -67.96727558581105200, -9.488692052113647080, -7.038790429923468039 ) ) ;
#33701=CARTESIAN_POINT ( 'NONE',  ( -65.15079379074605015, -9.165714244539783451, 1.521991683921744887 ) ) ;
#33703=CARTESIAN_POINT ( 'NONE',  ( -69.15027346225275551, -10.43622021222418716, -7.497281464624098390 ) ) ;
#33704=EDGE_LOOP ( 'NONE', ( #53360, #39019, #3590, #35321 ) ) ;
#33706=VERTEX_POINT ( 'NONE', #19915 ) ;
#33713=VECTOR ( 'NONE', #8711, 1000.000000000000114 ) ;
#33718=CARTESIAN_POINT ( 'NONE',  ( -67.08386678843554307, -11.40049507478859603, -4.138470222184133185 ) ) ;
#33731=CARTESIAN_POINT ( 'NONE',  ( 0.000000000000000000, 2.000000000000000000, 0.000000000000000000 ) ) ;
#33760=CARTESIAN_POINT ( 'NONE',  ( -65.16688019966139223, -9.167558940675322177, 1.648866456817433823 ) ) ;
#33807=CARTESIAN_POINT ( 'NONE',  ( -68.69950585158439083, -0.6013238516280168255, 6.175865180864700044 ) ) ;
#33892=CARTESIAN_POINT ( 'NONE',  ( -69.85628739008400601, 2.000000000006432632, -7.520604412859268173 ) ) ;
#33980=DIRECTION ( 'NONE',  ( 0.000000000000000000, -5.782411586589354681E-16, 1.000000000000000000 ) ) ;
#34067=CARTESIAN_POINT ( 'NONE',  ( -66.04860918961693983, -9.268670510630919068, -5.126440291711352515 ) ) ;
#34107=CARTESIAN_POINT ( 'NONE',  ( -66.80765385348918528, -11.36882057637399512, -7.559434449094163178 ) ) ;
#34109=CARTESIAN_POINT ( 'NONE',  ( -68.08080254705713230, -5.290906601729261638E-14, 7.854170068342909872 ) ) ;
#34137=ORIENTED_EDGE ( 'NONE', *, *, #25740, .F. ) ;
#34195=CARTESIAN_POINT ( 'NONE',  ( -68.73712005124077962, 0.1329671457173686178, 5.608481661908657934 ) ) ;
#34196=ORIENTED_EDGE ( 'NONE', *, *, #34373, .F. ) ;
#34199=CARTESIAN_POINT ( 'NONE',  ( -67.09057908004916726, -0.6008667158328537816, -1.335442097082733870 ) ) ;
#34203=EDGE_CURVE ( 'NONE', #53459, #19068, #1321, .T. ) ;
#34210=CARTESIAN_POINT ( 'NONE',  ( -70.00259797851279586, 0.1329035588801656675, 7.501778215771297553 ) ) ;
#34217=ORIENTED_EDGE ( 'NONE', *, *, #55930, .T. ) ;
#34345=ORIENTED_EDGE ( 'NONE', *, *, #42339, .F. ) ;
#34355=ORIENTED_EDGE ( 'NONE', *, *, #44255, .F. ) ;
#34373=EDGE_CURVE ( 'NONE', #7084, #25458, #3353, .T. ) ;
#34380=CARTESIAN_POINT ( 'NONE',  ( -69.19586433673185866, 2.103352214621878602E-14, 7.932749270814285047 ) ) ;
#34390=ORIENTED_EDGE ( 'NONE', *, *, #26500, .T. ) ;
#34447=EDGE_CURVE ( 'NONE', #18, #22349, #56198, .T. ) ;
#34448=CARTESIAN_POINT ( 'NONE',  ( -68.95754730983136938, 2.000000000004385825, -6.247493715005127513 ) ) ;
#34469=ORIENTED_EDGE ( 'NONE', *, *, #1904, .F. ) ;
#34482=EDGE_CURVE ( 'NONE', #12427, #18417, #46493, .T. ) ;
#34503=CYLINDRICAL_SURFACE ( 'NONE', #2280, 0.2499999999999998612 ) ;
#34518=ADVANCED_FACE ( 'NONE', ( #27493 ), #27897, .F. ) ;
#34524=B_SPLINE_CURVE_WITH_KNOTS ( 'NONE', 3,
 ( #53796, #19437, #6392, #45842, #10919, #49262 ),
 .UNSPECIFIED., .F., .F.,
 ( 4, 2, 4 ),
 ( 0.000000000000000000, 0.5000000000000000000, 1.000000000000000000 ),
 .UNSPECIFIED. ) ;
#34564=CARTESIAN_POINT ( 'NONE',  ( -66.64009219722507282, -11.34960557684216020, -2.652841686095987139 ) ) ;
#34570=CARTESIAN_POINT ( 'NONE',  ( -69.43545830293986398, -9.790829293527439248, 7.501778215771295777 ) ) ;
#34591=EDGE_CURVE ( 'NONE', #18, #13860, #1906, .T. ) ;
#34621=ORIENTED_EDGE ( 'NONE', *, *, #52757, .T. ) ;
#34636=CARTESIAN_POINT ( 'NONE',  ( 0.09621548157177385596, -1.683565401097096181, -2.125000000000000444 ) ) ;
#34638=CARTESIAN_POINT ( 'NONE',  ( 0.000000000000000000, 0.000000000000000000, 0.000000000000000000 ) ) ;
#34643=AXIS2_PLACEMENT_3D ( 'NONE', #55077, #11884, #55331 ) ;
#34724=CARTESIAN_POINT ( 'NONE',  ( -69.24559741778114130, 0.1329209457098951275, 6.496570960379585813 ) ) ;
#34776=CIRCLE ( 'NONE', #52932, 6.000000000000001776 ) ;
#34862=CARTESIAN_POINT ( 'NONE',  ( 5.618093942130458096, -1.050357310661657939, 2.260478214906367800 ) ) ;
#34865=CARTESIAN_POINT ( 'NONE',  ( -67.55782011861325032, -8.435184460786505412, -3.909888324369926060 ) ) ;
#34990=AXIS2_PLACEMENT_3D ( 'NONE', #18561, #44133, #36726 ) ;
#35107=FACE_OUTER_BOUND ( 'NONE', #30433, .T. ) ;
#35151=CARTESIAN_POINT ( 'NONE',  ( -67.86783029729696182, -11.27546072583064785, -7.472022508502797145 ) ) ;
#35162=CARTESIAN_POINT ( 'NONE',  ( 5.520171279030146039, -1.061450403529338837, -2.502362106692468835 ) ) ;
#35177=CARTESIAN_POINT ( 'NONE',  ( -1.246832498358330099E-15, 2.000000000000000000, 0.000000000000000000 ) ) ;
#35178=B_SPLINE_CURVE_WITH_KNOTS ( 'NONE', 3,
 ( #22859, #52671, #9238, #26558 ),
 .UNSPECIFIED., .F., .F.,
 ( 4, 4 ),
 ( 0.3613060669372403777, 0.3753454237082048950 ),
 .UNSPECIFIED. ) ;
#35198=CARTESIAN_POINT ( 'NONE',  ( 5.515120863165694942, -1.062156740595928683, 2.500028430129012325 ) ) ;
#35260=DIRECTION ( 'NONE',  ( -0.05705673239519651330, 0.9983709377222391712, 2.351258244848514932E-16 ) ) ;
#35285=CARTESIAN_POINT ( 'NONE',  ( -69.33582967021771992, 1.350899166405607588, 7.487487041937091803 ) ) ;
#35297=ORIENTED_EDGE ( 'NONE', *, *, #24412, .F. ) ;
#35321=ORIENTED_EDGE ( 'NONE', *, *, #39879, .F. ) ;
#35340=CARTESIAN_POINT ( 'NONE',  ( -57.29829478218162109, -10.27834239552269757, 4.211285351864063224E-15 ) ) ;
#35355=DIRECTION ( 'NONE',  ( 0.000000000000000000, 1.000000000000000000, 0.000000000000000000 ) ) ;
#35427=CARTESIAN_POINT ( 'NONE',  ( -66.40965317132554446, 8.186939909977519321E-16, 1.512899686938069088 ) ) ;
#35492=CARTESIAN_POINT ( 'NONE',  ( 4.930947970565946470, -1.129146301979396139, -1.967953638240999670 ) ) ;
#35499=CIRCLE ( 'NONE', #38246, 6.000000000000001776 ) ;
#35576=CARTESIAN_POINT ( 'NONE',  ( 4.902479726011971906, 0.000000000000000000, 2.247047898273224931 ) ) ;
#35597=ORIENTED_EDGE ( 'NONE', *, *, #51491, .T. ) ;
#35618=CARTESIAN_POINT ( 'NONE',  ( -69.11683642851026832, -9.015837829197110409, 7.493101075386320531 ) ) ;
#35620=B_SPLINE_CURVE_WITH_KNOTS ( 'NONE', 3,
 ( #3603, #3337, #38234, #11279, #55554, #42232, #33433, #7292 ),
 .UNSPECIFIED., .F., .F.,
 ( 4, 2, 2, 4 ),
 ( 4.816871102115739456E-16, 0.0004770940840306825957, 0.0009541881680608834803, 0.001908376336121245676 ),
 .UNSPECIFIED. ) ;
#35672=ORIENTED_EDGE ( 'NONE', *, *, #14519, .F. ) ;
#35715=CARTESIAN_POINT ( 'NONE',  ( -67.56320601492518563, -0.9999999999999978906, -2.442027903730110250 ) ) ;
#35724=CYLINDRICAL_SURFACE ( 'NONE', #15926, 3.000000000000001332 ) ;
#35765=ORIENTED_EDGE ( 'NONE', *, *, #30444, .T. ) ;
#35796=CARTESIAN_POINT ( 'NONE',  ( 0.1285714285714296967, 2.000000000000000000, -5.998622290806041590 ) ) ;
#35821=CARTESIAN_POINT ( 'NONE',  ( -68.84267254591711094, -9.186009798224464618, -7.487678583014048428 ) ) ;
#35827=CYLINDRICAL_SURFACE ( 'NONE', #22412, 2.125000000000000000 ) ;
#35851=CARTESIAN_POINT ( 'NONE',  ( -66.21705755929110637, -11.30109441652609270, 6.550948917181726117 ) ) ;
#35902=CARTESIAN_POINT ( 'NONE',  ( -67.55782011861325032, -8.435184460786505412, -3.909888324369926060 ) ) ;
#35921=ADVANCED_FACE ( 'NONE', ( #45323 ), #23477, .F. ) ;
#35943=CARTESIAN_POINT ( 'NONE',  ( -66.99840443968177794, -8.772812340773230133, 3.326521589947848412 ) ) ;
#36007=CARTESIAN_POINT ( 'NONE',  ( -68.54039869480983782, 0.1329787028216394551, 5.224814904089852163 ) ) ;
#36023=CARTESIAN_POINT ( 'NONE',  ( -68.44026216309750055, -1.000000000000000444, 5.059064008999124340 ) ) ;
#36029=CARTESIAN_POINT ( 'NONE',  ( -69.22881859397718074, 1.437012684761762582, -7.485193420789064689 ) ) ;
#36048=ORIENTED_EDGE ( 'NONE', *, *, #31022, .F. ) ;
#36050=CARTESIAN_POINT ( 'NONE',  ( -67.47405682104675861, -8.826835280158354280, -4.659789304343650684 ) ) ;
#36083=CARTESIAN_POINT ( 'NONE',  ( -70.10169143752739274, -0.9999999999999995559, 7.503902134509972122 ) ) ;
#36096=CARTESIAN_POINT ( 'NONE',  ( 5.515141197255969630, -1.062154408800312755, -2.500037664106760094 ) ) ;
#36136=CARTESIAN_POINT ( 'NONE',  ( -67.25395622669698525, -9.540674738394741894, 3.391838660562430441 ) ) ;
#36140=CARTESIAN_POINT ( 'NONE',  ( -67.39372447183772863, -4.296715151703168435E-12, 4.869406872007187914 ) ) ;
#36152=DIRECTION ( 'NONE',  ( -0.000000000000000000, -1.000000000000000000, -0.000000000000000000 ) ) ;
#36202=CARTESIAN_POINT ( 'NONE',  ( -67.50810339439870233, 2.000000000000000000, 7.448312483692316022 ) ) ;
#36225=CARTESIAN_POINT ( 'NONE',  ( -66.74449147233332269, -11.36157748060019301, 7.448312483692313357 ) ) ;
#36251=CARTESIAN_POINT ( 'NONE',  ( 4.912750499197525045, -1.131233082521085231, 2.061810099490657411 ) ) ;
#36261=CARTESIAN_POINT ( 'NONE',  ( -68.12990498669439887, 0.1329617757551050938, 4.288727116335238954 ) ) ;
#36263=B_SPLINE_CURVE_WITH_KNOTS ( 'NONE', 3,
 ( #13704, #53196, #10293, #10599, #23078, #9453, #49180, #31321, #13994, #27914, #45218, #26777, #44101, #5216, #22528, #52883 ),
 .UNSPECIFIED., .F., .F.,
 ( 4, 2, 2, 2, 2, 2, 2, 4 ),
 ( 3.469446951953613804E-18, 0.001965516910292332883, 0.003931033820584662296, 0.007862067641169319387, 0.009827584551461647500, 0.01179310146175397735, 0.01375861837204630372, 0.01572413528233863184 ),
 .UNSPECIFIED. ) ;
#36276=CARTESIAN_POINT ( 'NONE',  ( -70.11839600776268355, -1.000000000000000666, -7.555920072494595630 ) ) ;
#36304=DIRECTION ( 'NONE',  ( -0.05705673239519651330, 0.9983709377222391712, 2.351258244848514932E-16 ) ) ;
#36334=EDGE_CURVE ( 'NONE', #3029, #44205, #16018, .T. ) ;
#36385=CARTESIAN_POINT ( 'NONE',  ( -68.36693371783928797, -11.54762975344078768, 6.564485215144721941 ) ) ;
#36390=CARTESIAN_POINT ( 'NONE',  ( -67.85140231345076245, -4.690475086145005873E-12, -5.859509639698581296 ) ) ;
#36407=CARTESIAN_POINT ( 'NONE',  ( -69.51265309394176484, -9.414302016845754295, -7.502502568033363239 ) ) ;
#36426=CARTESIAN_POINT ( 'NONE',  ( -69.66297551618575312, -8.676591480033549075, 7.503902134509970345 ) ) ;
#36445=ORIENTED_EDGE ( 'NONE', *, *, #32733, .F. ) ;
#36459=CARTESIAN_POINT ( 'NONE',  ( -67.32595136268157887, -0.9999999999999974465, 0.5932824550257459473 ) ) ;
#36485=CARTESIAN_POINT ( 'NONE',  ( -67.30928982028858343, -11.38498548360074025, 7.460396425438591272 ) ) ;
#36486=ORIENTED_EDGE ( 'NONE', *, *, #45911, .F. ) ;
#36511=CARTESIAN_POINT ( 'NONE',  ( 0.1285714285714289751, 0.000000000000000000, -5.998622290806042479 ) ) ;
#36548=CARTESIAN_POINT ( 'NONE',  ( -69.79279777665210815, 0.8065827901120606880, -7.497281464624094838 ) ) ;
#36557=ORIENTED_EDGE ( 'NONE', *, *, #9239, .T. ) ;
#36562=EDGE_CURVE ( 'NONE', #37474, #27104, #9888, .T. ) ;
#36566=CIRCLE ( 'NONE', #28406, 2.125000000000000000 ) ;
#36599=AXIS2_PLACEMENT_3D ( 'NONE', #33731, #50211, #49923 ) ;
#36634=VECTOR ( 'NONE', #49027, 1000.000000000000114 ) ;
#36636=CARTESIAN_POINT ( 'NONE',  ( 5.417481111513990477, -1.073353501383011110, -2.423381879925703419 ) ) ;
#36668=ORIENTED_EDGE ( 'NONE', *, *, #14519, .T. ) ;
#36680=CARTESIAN_POINT ( 'NONE',  ( -68.36638157653975156, 9.462817827437976943E-12, -6.792143739499517885 ) ) ;
#36726=DIRECTION ( 'NONE',  ( -0.9090593428863094072, 0.000000000000000000, 0.4166666666666669072 ) ) ;
#36740=FILL_AREA_STYLE_COLOUR ( '', #9292 ) ;
#36775=AXIS2_PLACEMENT_3D ( 'NONE', #45607, #41072, #19496 ) ;
#36795=VERTEX_POINT ( 'NONE', #2575 ) ;
#36818=LINE ( 'NONE', #54134, #3853 ) ;
#36879=CARTESIAN_POINT ( 'NONE',  ( -66.93067463247570004, -9.369820663055195453, 6.899827505725927068 ) ) ;
#36884=CARTESIAN_POINT ( 'NONE',  ( 5.454592090961234874, -6.230699628392517120, -2.061810099490657411 ) ) ;
#36950=CARTESIAN_POINT ( 'NONE',  ( 5.284044854955649129, -1.088655197871726710, 2.393421119419573806 ) ) ;
#36971=CARTESIAN_POINT ( 'NONE',  ( -66.51077781314475601, -11.33477655279809326, 1.402349447197485777 ) ) ;
#36975=CARTESIAN_POINT ( 'NONE',  ( -66.44888886210301848, -1.718375678206839771E-11, -0.7138195548296715209 ) ) ;
#36998=ORIENTED_EDGE ( 'NONE', *, *, #25020, .F. ) ;
#37043=CARTESIAN_POINT ( 'NONE',  ( -70.06496498987883115, 0.1329914806336913169, 7.577667541101601678 ) ) ;
#37077=EDGE_LOOP ( 'NONE', ( #4484, #31760, #23724, #48306 ) ) ;
#37136=CARTESIAN_POINT ( 'NONE',  ( -66.63077082645354210, -8.730603027686937523, 1.362417606690507377 ) ) ;
#37182=EDGE_CURVE ( 'NONE', #8945, #7825, #31509, .T. ) ;
#37194=CARTESIAN_POINT ( 'NONE',  ( -67.13303327250461905, 2.471980953266950741E-14, 6.321089406856109427 ) ) ;
#37220=CARTESIAN_POINT ( 'NONE',  ( -65.61040098691356093, 2.602085213965210642E-15, 0.7610157271807490575 ) ) ;
#37231=ADVANCED_FACE ( 'NONE', ( #48116 ), #34503, .T. ) ;
#37264=EDGE_CURVE ( 'NONE', #13853, #39622, #48543, .T. ) ;
#37290=CARTESIAN_POINT ( 'NONE',  ( -67.11631774061213207, 2.000000000000002220, 0.4315550088921883409 ) ) ;
#37374=CARTESIAN_POINT ( 'NONE',  ( -69.35974691127840686, -9.648372592778560630, -8.803577518029834792 ) ) ;
#37391=CARTESIAN_POINT ( 'NONE',  ( -64.63669322539915640, -11.11986739470662933, 1.314563741827290189 ) ) ;
#37396=CARTESIAN_POINT ( 'NONE',  ( -66.56540940824446295, -9.327934164263727013, 6.231849021620877060 ) ) ;
#37472=CIRCLE ( 'NONE', #30241, 2.125000000000000000 ) ;
#37474=VERTEX_POINT ( 'NONE', #36202 ) ;
#37499=CARTESIAN_POINT ( 'NONE',  ( -69.19091591890759219, -11.64211925634823608, -7.659292557883813579 ) ) ;
#37573=VECTOR ( 'NONE', #7635, 1000.000000000000114 ) ;
#37594=CARTESIAN_POINT ( 'NONE',  ( -67.02251838831884356, -0.6010030055608566180, -0.3300946888591886896 ) ) ;
#37609=CARTESIAN_POINT ( 'NONE',  ( -68.96274401086908767, -10.65449282557018584, 7.493821216008848651 ) ) ;
#37669=( BOUNDED_CURVE ( )  B_SPLINE_CURVE ( 3, ( #41363, #2452, #45893, #19773 ),
 .UNSPECIFIED., .F., .F. ) 
 B_SPLINE_CURVE_WITH_KNOTS ( ( 4, 4 ),
 ( -8.881784197001252323E-16, 0.3848561846235226125 ),
 .UNSPECIFIED. ) 
 CURVE ( )  GEOMETRIC_REPRESENTATION_ITEM ( )  RATIONAL_B_SPLINE_CURVE ( ( 1.000000000000000000, 0.9876951826469675400, 0.9876951826469675400, 1.000000000000000000 ) ) 
 REPRESENTATION_ITEM ( '' )  );
#37678=LINE ( 'NONE', #45096, #19121 ) ;
#37696=DIRECTION ( 'NONE',  ( -0.9090593428863091852, 0.000000000000000000, -0.4166666666666674623 ) ) ;
#37704=CARTESIAN_POINT ( 'NONE',  ( -65.54552266609172761, -11.22408668727510239, -5.120420914815952962 ) ) ;
#37708=CARTESIAN_POINT ( 'NONE',  ( -68.22482764337692629, -9.518226629270689187, 7.369622379056326444 ) ) ;
#37753=ORIENTED_EDGE ( 'NONE', *, *, #38437, .T. ) ;
#37759=ADVANCED_FACE ( 'NONE', ( #55887 ), #10131, .F. ) ;
#37811=CARTESIAN_POINT ( 'NONE',  ( -68.37651787278942095, 7.120427645301669091E-12, 6.778377825370101029 ) ) ;
#37870=CARTESIAN_POINT ( 'NONE',  ( -69.48902198128583052, 0.1329003158168008403, 6.824617610603328721 ) ) ;
#37881=CYLINDRICAL_SURFACE ( 'NONE', #30732, 3.000000000000001332 ) ;
#37885=CARTESIAN_POINT ( 'NONE',  ( -67.35931108517087296, 1.999999999999983569, -7.222001337324623904 ) ) ;
#37888=CARTESIAN_POINT ( 'NONE',  ( -67.46543143576477064, -0.6008375282045697041, 3.326521589947856405 ) ) ;
#37895=VERTEX_POINT ( 'NONE', #4751 ) ;
#37982=CARTESIAN_POINT ( 'NONE',  ( -65.90632570267226242, -9.252354265052927573, 0.3563396981035996669 ) ) ;
#37985=CARTESIAN_POINT ( 'NONE',  ( -69.40690260994486493, -9.931727281594525891, -7.501514206501486370 ) ) ;
#37994=DIRECTION ( 'NONE',  ( 0.000000000000000000, -0.000000000000000000, -1.000000000000000000 ) ) ;
#37996=( BOUNDED_CURVE ( )  B_SPLINE_CURVE ( 3, ( #8197, #20704, #29795, #42821 ),
 .UNSPECIFIED., .F., .F. ) 
 B_SPLINE_CURVE_WITH_KNOTS ( ( 4, 4 ),
 ( 3.141592653589797113, 4.281995669727205467 ),
 .UNSPECIFIED. ) 
 CURVE ( )  GEOMETRIC_REPRESENTATION_ITEM ( )  RATIONAL_B_SPLINE_CURVE ( ( 1.000000000000000000, 0.8945281452387652266, 0.8945281452387652266, 1.000000000000000000 ) ) 
 REPRESENTATION_ITEM ( '' )  );
#37998=CARTESIAN_POINT ( 'NONE',  ( -69.67957132394272435, -8.678494591075715192, -7.555920072494596518 ) ) ;
#38024=FACE_BOUND ( 'NONE', #12369, .T. ) ;
#38035=CARTESIAN_POINT ( 'NONE',  ( -65.08325356666762218, -9.157969123114190424, 0.6641167203970371746 ) ) ;
#38054=CARTESIAN_POINT ( 'NONE',  ( 5.454592090961233097, -6.230699628392518008, 2.061810099490656079 ) ) ;
#38055=CARTESIAN_POINT ( 'NONE',  ( 0.1285714285714296967, 2.000000000000000000, -5.998622290806041590 ) ) ;
#38078=CARTESIAN_POINT ( 'NONE',  ( 0.2239497891030736432, -1.668917571073590400, 5.998622290806041590 ) ) ;
#38121=FACE_BOUND ( 'NONE', #45636, .T. ) ;
#38134=CARTESIAN_POINT ( 'NONE',  ( -58.00000000000000711, 2.000000000000000000, 7.102951435054649637E-15 ) ) ;
#38139=CARTESIAN_POINT ( 'NONE',  ( -68.27330710698295491, 2.000000000000001332, -8.536061506181777503 ) ) ;
#38142=CARTESIAN_POINT ( 'NONE',  ( -69.10252959121689287, -0.6012852789374203422, 6.810182420670475523 ) ) ;
#38195=CARTESIAN_POINT ( 'NONE',  ( 5.488878199366571842, 0.000000000000000000, -2.420139938591586493 ) ) ;
#38219=CARTESIAN_POINT ( 'NONE',  ( -65.88104832801796817, -9.249455602226623441, 1.512899686938066868 ) ) ;
#38234=CARTESIAN_POINT ( 'NONE',  ( -69.33786762168887208, -0.4146581964375588014, 7.487530722355575818 ) ) ;
#38246=AXIS2_PLACEMENT_3D ( 'NONE', #17781, #48130, #8133 ) ;
#38254=FACE_BOUND ( 'NONE', #46490, .T. ) ;
#38255=CARTESIAN_POINT ( 'NONE',  ( -68.45082166678818680, -0.05101588947699599308, -7.468518229136111408 ) ) ;
#38257=CARTESIAN_POINT ( 'NONE',  ( -68.50231803695028532, -8.543494007632165932, -5.847034362371243965 ) ) ;
#38278=EDGE_CURVE ( 'NONE', #17419, #32512, #42830, .T. ) ;
#38302=CARTESIAN_POINT ( 'NONE',  ( -65.06940864783059908, -9.156381468068820695, -0.6466721865750668652 ) ) ;
#38321=DIRECTION ( 'NONE',  ( -0.05705673239519651330, 0.9983709377222391712, 2.351258244848514932E-16 ) ) ;
#38343=CARTESIAN_POINT ( 'NONE',  ( -67.84662069460095779, -4.914479465932832227E-13, 5.846634436083241404 ) ) ;
#38403=CARTESIAN_POINT ( 'NONE',  ( 0.3240706152708093812, -3.670543518250628967, -1.335466778558061241E-15 ) ) ;
#38424=CARTESIAN_POINT ( 'NONE',  ( -67.63293690793081225, 0.1329915468650123000, 2.735910648338365725 ) ) ;
#38437=EDGE_CURVE ( 'NONE', #32717, #9189, #15702, .T. ) ;
#38509=CARTESIAN_POINT ( 'NONE',  ( -70.27375990177029053, -9.753186304793430850, -9.798907322976864620 ) ) ;
#38541=CARTESIAN_POINT ( 'NONE',  ( 4.930947970565944694, -1.129146301979397693, 1.967953638241001446 ) ) ;
#38586=CIRCLE ( 'NONE', #7735, 2.125000000000000000 ) ;
#38662=B_SPLINE_CURVE_WITH_KNOTS ( 'NONE', 3,
 ( #48970, #26544, #23142, #23425, #1562, #52655, #49244, #27117, #18594, #44167, #1809, #53260, #10358, #22308, #26842, #5271, #35943, #14354, #45010, #18888, #6121, #31667, #40471, #53507, #30816, #22581, #970, #44422 ),
 .UNSPECIFIED., .F., .F.,
 ( 4, 2, 2, 2, 2, 2, 2, 2, 2, 2, 2, 2, 2, 4 ),
 ( 7.806255641895624221E-18, 0.002014507434814107479, 0.004029014869628207152, 0.006043522304442306391, 0.007050776021849359046, 0.008058029739256412569, 0.009065283456663466091, 0.01007253717407051788, 0.01208704460888462319, 0.01309429832629167845, 0.01410155204369873023, 0.01510880576110578376, 0.01561243261980931225, 0.01611605947851283901 ),
 .UNSPECIFIED. ) ;
#38702=ADVANCED_FACE ( 'NONE', ( #4900 ), #685, .F. ) ;
#38719=VECTOR ( 'NONE', #28501, 1000.000000000000000 ) ;
#38723=CARTESIAN_POINT ( 'NONE',  ( 5.211213849286742139, 0.000000000000000000, -2.388555951666874844 ) ) ;
#38733=CARTESIAN_POINT ( 'NONE',  ( -66.79351738431421381, 1.999999999999980460, 6.196202711026808529 ) ) ;
#38753=ORIENTED_EDGE ( 'NONE', *, *, #36562, .F. ) ;
#38768=ORIENTED_EDGE ( 'NONE', *, *, #28373, .T. ) ;
#38848=CARTESIAN_POINT ( 'NONE',  ( -66.90530812237336988, -8.360358167099663618, 0.5932824550257441709 ) ) ;
#38873=CARTESIAN_POINT ( 'NONE',  ( 0.2239497891030733101, -1.668917571073584627, -5.998622290806041590 ) ) ;
#38874=CARTESIAN_POINT ( 'NONE',  ( -67.92407581255017135, -9.617479462011470304, -5.273316683197693422 ) ) ;
#38876=ORIENTED_EDGE ( 'NONE', *, *, #26500, .F. ) ;
#38879=VECTOR ( 'NONE', #12857, 1000.000000000000000 ) ;
#38895=CARTESIAN_POINT ( 'NONE',  ( -66.57831216173161692, 3.903127820947815962E-15, -5.126440291711408470 ) ) ;
#38960=CARTESIAN_POINT ( 'NONE',  ( -69.11683642851026832, -9.015837829197110409, 7.493101075386320531 ) ) ;
#38995=CARTESIAN_POINT ( 'NONE',  ( -66.76709096105220453, 1.999999999999983569, -6.184885810276858464 ) ) ;
#39019=ORIENTED_EDGE ( 'NONE', *, *, #23025, .F. ) ;
#39105=CARTESIAN_POINT ( 'NONE',  ( 4.848100717410752658, 0.000000000000000000, 2.029539223447463847 ) ) ;
#39155=CARTESIAN_POINT ( 'NONE',  ( 5.221828392167460642, 0.000000000000000000, -2.393421119419572918 ) ) ;
#39175=CARTESIAN_POINT ( 'NONE',  ( 0.3240706152708103804, -3.670543518250629855, 2.124999999999998668 ) ) ;
#39204=ORIENTED_EDGE ( 'NONE', *, *, #21987, .F. ) ;
#39248=B_SPLINE_CURVE_WITH_KNOTS ( 'NONE', 1,
 ( #34210, #4087 ),
 .UNSPECIFIED., .F., .F.,
 ( 2, 2 ),
 ( 0.001874228446202061112, 0.003011459512596941206 ),
 .UNSPECIFIED. ) ;
#39324=CARTESIAN_POINT ( 'NONE',  ( 0.4518049228021099872, -3.655895688227116747, -5.998622290806042479 ) ) ;
#39358=ORIENTED_EDGE ( 'NONE', *, *, #42262, .T. ) ;
#39406=ORIENTED_EDGE ( 'NONE', *, *, #30027, .T. ) ;
#39445=ADVANCED_FACE ( 'NONE', ( #6652 ), #4653, .T. ) ;
#39453=CYLINDRICAL_SURFACE ( 'NONE', #52740, 0.2499999999999998612 ) ;
#39501=( BOUNDED_CURVE ( )  B_SPLINE_CURVE ( 3, ( #21584, #56201, #30665, #39155 ),
 .UNSPECIFIED., .F., .F. ) 
 B_SPLINE_CURVE_WITH_KNOTS ( ( 4, 4 ),
 ( 3.528432781240732563, 5.142782291042179210 ),
 .UNSPECIFIED. ) 
 CURVE ( )  GEOMETRIC_REPRESENTATION_ITEM ( )  RATIONAL_B_SPLINE_CURVE ( ( 1.000000000000000000, 0.7943613114863588009, 0.7943613114863588009, 1.000000000000000000 ) ) 
 REPRESENTATION_ITEM ( '' )  );
#39536=CARTESIAN_POINT ( 'NONE',  ( 0.000000000000000000, 0.000000000000000000, 0.000000000000000000 ) ) ;
#39561=CARTESIAN_POINT ( 'NONE',  ( 4.912750499197525933, -1.131233082521086342, 2.029539223447463403 ) ) ;
#39576=CARTESIAN_POINT ( 'NONE',  ( -69.43561177275644525, -9.791245164465275153, -7.501782499249458169 ) ) ;
#39622=VERTEX_POINT ( 'NONE', #15640 ) ;
#39635=DIRECTION ( 'NONE',  ( -0.9983709377222390602, -0.05705673239519638146, 0.000000000000000000 ) ) ;
#39682=CARTESIAN_POINT ( 'NONE',  ( 4.966775449259088759, -1.125037814383460288, 2.247047898273225375 ) ) ;
#39699=CYLINDRICAL_SURFACE ( 'NONE', #45594, 2.125000000000000000 ) ;
#39747=ORIENTED_EDGE ( 'NONE', *, *, #27467, .F. ) ;
#39879=EDGE_CURVE ( 'NONE', #48284, #43429, #40032, .T. ) ;
#39946=CARTESIAN_POINT ( 'NONE',  ( 4.848100717410752658, 0.000000000000000000, 2.061810099490657411 ) ) ;
#40032=LINE ( 'NONE', #17920, #42859 ) ;
#40050=CARTESIAN_POINT ( 'NONE',  ( -57.52614991588065152, -8.291364278369167451, 5.150256511358686722E-15 ) ) ;
#40138=MECHANICAL_DESIGN_GEOMETRIC_PRESENTATION_REPRESENTATION('',(#25623),#41028);
#40177=DIRECTION ( 'NONE',  ( 0.9031405107545329436, 0.1035669190568594411, -0.4166666666666669072 ) ) ;
#40181=AXIS2_PLACEMENT_3D ( 'NONE', #8758, #7602, #3050 ) ;
#40217=EDGE_CURVE ( 'NONE', #17834, #13134, #37996, .T. ) ;
#40229=CARTESIAN_POINT ( 'NONE',  ( 0.1285714285714296967, 2.000000000000000000, -5.998622290806041590 ) ) ;
#40245=CARTESIAN_POINT ( 'NONE',  ( -70.83115287062283016, -1.183819181302419339E-15, -9.798907322976862844 ) ) ;
#40316=CARTESIAN_POINT ( 'NONE',  ( -67.98273966911209243, -0.9999999999999983347, -3.909888324369924284 ) ) ;
#40349=CARTESIAN_POINT ( 'NONE',  ( -67.91473901113046452, -9.431317234435587338, -7.468518229136111408 ) ) ;
#40381=CARTESIAN_POINT ( 'NONE',  ( -66.78520713108927964, -9.487000657996272679, 0.6944083025908609486 ) ) ;
#40385=CARTESIAN_POINT ( 'NONE',  ( -65.67461282944442758, 2.602085213965210642E-15, 1.521991683923406224 ) ) ;
#40444=VECTOR ( 'NONE', #11112, 1000.000000000000114 ) ;
#40471=CARTESIAN_POINT ( 'NONE',  ( -68.35070498065327627, -8.927360579512033212, 6.387117138744199174 ) ) ;
#40486=CARTESIAN_POINT ( 'NONE',  ( 5.850167541230363533, 0.0001172166011806737484, 1.544991542362377901 ) ) ;
#40543=B_SPLINE_SURFACE_WITH_KNOTS ( 'NONE', 1, 3, ( 
 ( #11741, #19134, #27967, #49807, #46102, #6945, #10905, #37290, #28800, #23960, #54599, #41567, #16017, #29058 ),
 ( #41293, #28216, #33342, #45528, #46359, #7474, #6648, #36459, #53776, #32222, #45274, #40998, #2386, #54341 ) ),
 .UNSPECIFIED., .F., .F., .F.,
 ( 2, 2 ),
 ( 4, 2, 2, 2, 2, 2, 4 ),
 ( 0.000000000000000000, 1.000000000000000000 ),
 ( 0.000000000000000000, 0.1159099261691615840, 0.2318198523383231680, 0.4636397046766463359, 0.6954595570149695316, 0.9272794093532926718, 1.000000000000000000 ),
 .UNSPECIFIED. ) ;
#40580=CARTESIAN_POINT ( 'NONE',  ( -66.86496996703597517, -9.362286032850320794, -4.884162593219725679 ) ) ;
#40600=B_SPLINE_CURVE_WITH_KNOTS ( 'NONE', 3,
 ( #3779, #16029, #33058, #12016 ),
 .UNSPECIFIED., .F., .F.,
 ( 4, 4 ),
 ( 0.6246544700140113093, 0.6386939402607147986 ),
 .UNSPECIFIED. ) ;
#40630=ORIENTED_EDGE ( 'NONE', *, *, #30197, .F. ) ;
#40669=CARTESIAN_POINT ( 'NONE',  ( -67.85651025736190434, -11.48909734946287386, 5.667235587292936749 ) ) ;
#40673=CARTESIAN_POINT ( 'NONE',  ( -69.19654577526263495, 4.553649124439119412E-15, -7.934121704141924525 ) ) ;
#40707=CARTESIAN_POINT ( 'NONE',  ( -66.90530812237336988, -8.360358167099661841, 0.5932824550257441709 ) ) ;
#40756=DIRECTION ( 'NONE',  ( 0.000000000000000000, -1.000000000000000000, 0.000000000000000000 ) ) ;
#40868=CARTESIAN_POINT ( 'NONE',  ( -67.56320601492518563, -0.9999999999999978906, -2.442027903730110250 ) ) ;
#40921=CARTESIAN_POINT ( 'NONE',  ( -69.49740922963668766, -9.798021964684151541, 7.577667541101590132 ) ) ;
#40925=CARTESIAN_POINT ( 'NONE',  ( -69.23745231081454676, -0.5995258673811661998, -7.041125024142530719 ) ) ;
#40927=DIRECTION ( 'NONE',  ( -0.1139275668495183524, 0.9934890585767659488, 4.694855797473114533E-16 ) ) ;
#40984=CARTESIAN_POINT ( 'NONE',  ( -67.27849890436391433, -9.409707134521932304, 7.454917401049827141 ) ) ;
#40991=ORIENTED_EDGE ( 'NONE', *, *, #46205, .F. ) ;
#40998=CARTESIAN_POINT ( 'NONE',  ( -70.38892378062969613, -1.000000000000148992, 7.852029984319922384 ) ) ;
#41007=CIRCLE ( 'NONE', #36599, 2.125000000000000000 ) ;
#41028=( GEOMETRIC_REPRESENTATION_CONTEXT ( 3 ) GLOBAL_UNCERTAINTY_ASSIGNED_CONTEXT ( ( #47265 ) ) GLOBAL_UNIT_ASSIGNED_CONTEXT ( ( #45508, #41273, #27102 ) ) REPRESENTATION_CONTEXT ( 'NONE', 'WORKASPACE' ) );
#41072=DIRECTION ( 'NONE',  ( 0.000000000000000000, 1.000000000000000000, 0.000000000000000000 ) ) ;
#41112=CARTESIAN_POINT ( 'NONE',  ( -67.82503658922976797, -9.472380908384517184, -6.792143739504113320 ) ) ;
#41113=EDGE_CURVE ( 'NONE', #46706, #13860, #34776, .T. ) ;
#41143=CARTESIAN_POINT ( 'NONE',  ( 0.09621548157177266247, -1.683565401097097070, -3.964956190634384326E-16 ) ) ;
#41213=CARTESIAN_POINT ( 'NONE',  ( -68.53751928918664760, 4.336808689942017736E-15, -8.456585623303165988 ) ) ;
#41220=DIRECTION ( 'NONE',  ( 0.9997703818010067467, -0.000000000000000000, -0.02142857142857158143 ) ) ;
#41273=( NAMED_UNIT ( * ) PLANE_ANGLE_UNIT ( ) SI_UNIT ( $, .RADIAN. ) );
#41293=CARTESIAN_POINT ( 'NONE',  ( -71.01620612404938981, -1.000000000000001332, -8.550077602493738382 ) ) ;
#41363=CARTESIAN_POINT ( 'NONE',  ( 4.848100717410754434, 0.000000000000000000, -2.061810099490656079 ) ) ;
#41388=CARTESIAN_POINT ( 'NONE',  ( -70.57153585115312922, -8.780779913117140012, -8.550077602493740159 ) ) ;
#41408=CARTESIAN_POINT ( 'NONE',  ( -65.08700002776164695, -9.158398745557436271, 0.7610157271824009584 ) ) ;
#41427=FACE_OUTER_BOUND ( 'NONE', #10163, .T. ) ;
#41474=CARTESIAN_POINT ( 'NONE',  ( -66.34686992624823176, -1.387778780781445676E-14, 4.515874129472569720 ) ) ;
#41503=CARTESIAN_POINT ( 'NONE',  ( -65.59336848870630376, 4.336808689942017736E-15, -0.3798655365425420150 ) ) ;
#41532=ORIENTED_EDGE ( 'NONE', *, *, #39879, .T. ) ;
#41542=PLANE ( 'NONE',  #54022 ) ;
#41567=CARTESIAN_POINT ( 'NONE',  ( -70.12629345720861807, 1.999999999999801048, 7.856885134693458284 ) ) ;
#41655=CARTESIAN_POINT ( 'NONE',  ( -64.77372111108157071, -11.13558095840576989, -2.612833193081008698 ) ) ;
#41659=CARTESIAN_POINT ( 'NONE',  ( -65.38822204059790977, -9.192941140068732864, 3.032081494020515411 ) ) ;
#41702=PLANE ( 'NONE',  #34643 ) ;
#41750=CARTESIAN_POINT ( 'NONE',  ( -68.87570450778353859, -0.6013635744588955445, 6.466593069172607677 ) ) ;
#41753=DIRECTION ( 'NONE',  ( 2.551063935260010306E-17, -4.081702296416016490E-16, 1.000000000000000000 ) ) ;
#41782=ORIENTED_EDGE ( 'NONE', *, *, #25224, .T. ) ;
#41826=CARTESIAN_POINT ( 'NONE',  ( -58.00000000000000711, 2.000000000000000000, 3.000000000000008438 ) ) ;
#41827=CARTESIAN_POINT ( 'NONE',  ( -67.27849890436391433, -9.409707134521932304, 7.454917401049827141 ) ) ;
#41839=CARTESIAN_POINT ( 'NONE',  ( 5.912796793901486048, -6.204513306124834315, -2.260536671351835558 ) ) ;
#41840=B_SPLINE_CURVE_WITH_KNOTS ( 'NONE', 1,
 ( #53407, #14780 ),
 .UNSPECIFIED., .F., .F.,
 ( 2, 2 ),
 ( 2.168404344971008627E-19, 0.0006430183911724570312 ),
 .UNSPECIFIED. ) ;
#41921=LINE ( 'NONE', #29451, #44719 ) ;
#41933=CARTESIAN_POINT ( 'NONE',  ( -67.01030352016741176, -8.774176600361034417, 3.370402386379092619 ) ) ;
#41946=LINE ( 'NONE', #55045, #48475 ) ;
#42033=CARTESIAN_POINT ( 'NONE',  ( -58.00000000000000711, 2.000000000000000000, 7.102951435054649637E-15 ) ) ;
#42061=ORIENTED_EDGE ( 'NONE', *, *, #49291, .F. ) ;
#42123=CARTESIAN_POINT ( 'NONE',  ( -69.14139375802285770, 2.000000000002681855, -6.539696485998404363 ) ) ;
#42146=CARTESIAN_POINT ( 'NONE',  ( -68.63426800804415961, -10.92493131198209078, 7.487487041937088250 ) ) ;
#42213=CARTESIAN_POINT ( 'NONE',  ( -70.57579075201010710, -8.781267840485488918, 8.554889286408839055 ) ) ;
#42215=EDGE_CURVE ( 'NONE', #25458, #33250, #12793, .T. ) ;
#42228=ORIENTED_EDGE ( 'NONE', *, *, #53223, .F. ) ;
#42232=CARTESIAN_POINT ( 'NONE',  ( -68.45424121227161152, -0.05181598292322161375, 7.468591521940118660 ) ) ;
#42239=CARTESIAN_POINT ( 'NONE',  ( -66.08148974733411762, -11.28554828561908074, -6.315096454939365778 ) ) ;
#42243=CARTESIAN_POINT ( 'NONE',  ( -65.14865909603261684, -9.165469450123071127, -1.520040349670753743 ) ) ;
#42254=PLANE ( 'NONE',  #47581 ) ;
#42262=EDGE_CURVE ( 'NONE', #16329, #21409, #41946, .T. ) ;
#42339=EDGE_CURVE ( 'NONE', #3658, #22349, #3349, .T. ) ;
#42345=CARTESIAN_POINT ( 'NONE',  ( -68.36985609944017028, -0.6011933878353118432, 5.577208301935089096 ) ) ;
#42355=ORIENTED_EDGE ( 'NONE', *, *, #16323, .T. ) ;
#42385=ADVANCED_FACE ( 'NONE', ( #13823 ), #47107, .T. ) ;
#42391=VECTOR ( 'NONE', #15722, 1000.000000000000114 ) ;
#42395=DIRECTION ( 'NONE',  ( 0.000000000000000000, 5.782411586589354681E-16, -1.000000000000000000 ) ) ;
#42421=CARTESIAN_POINT ( 'NONE',  ( -66.43251979230488757, 1.999999999999989120, -5.460169066007572347 ) ) ;
#42467=CYLINDRICAL_SURFACE ( 'NONE', #5856, 2.125000000000000000 ) ;
#42496=CARTESIAN_POINT ( 'NONE',  ( -70.26988861484534254, -8.746188756442855095, 8.208045577613539479 ) ) ;
#42518=CARTESIAN_POINT ( 'NONE',  ( -65.31815034969253020, -11.19801294790904578, -4.498572511313247979 ) ) ;
#42520=ORIENTED_EDGE ( 'NONE', *, *, #13029, .F. ) ;
#42521=CARTESIAN_POINT ( 'NONE',  ( -67.14859018435215887, -9.394809955489860087, 5.522897687430004865 ) ) ;
#42533=CARTESIAN_POINT ( 'NONE',  ( -69.06076127825900812, -0.2533158072296424201, -7.481591365497656021 ) ) ;
#42536=CARTESIAN_POINT ( 'NONE',  ( -67.41690247247410639, -11.43868567671724890, 4.989023737097910249 ) ) ;
#42569=CARTESIAN_POINT ( 'NONE',  ( -65.44866277073604977, -9.199872132678805770, 3.266248677641420350 ) ) ;
#42581=EDGE_LOOP ( 'NONE', ( #56024, #44381, #7129, #47769 ) ) ;
#42585=ORIENTED_EDGE ( 'NONE', *, *, #19840, .F. ) ;
#42594=CARTESIAN_POINT ( 'NONE',  ( -69.76593803006062444, -0.7338954340007644017, -7.496705766434927476 ) ) ;
#42604=CARTESIAN_POINT ( 'NONE',  ( -68.19194133488814202, 5.005647646799308669E-13, 6.473804834635568994 ) ) ;
#42607=DIRECTION ( 'NONE',  ( -0.4165485852472824990, -0.02380568209675230223, 0.9088017196442774726 ) ) ;
#42617=ORIENTED_EDGE ( 'NONE', *, *, #50262, .T. ) ;
#42638=ORIENTED_EDGE ( 'NONE', *, *, #9306, .F. ) ;
#42658=CARTESIAN_POINT ( 'NONE',  ( -67.79361442428482576, 2.000000000000000000, 7.454431982338135754 ) ) ;
#42664=CARTESIAN_POINT ( 'NONE',  ( 0.1285714285714296967, 2.000000000000000000, -5.998622290806041590 ) ) ;
#42674=CARTESIAN_POINT ( 'NONE',  ( -66.45493427417522980, 1.999999999999980460, 5.466724623769072977 ) ) ;
#42723=DIRECTION ( 'NONE',  ( 0.05705673239519650636, -0.9983709377222390602, -2.328121953249066419E-16 ) ) ;
#42725=PRODUCT_DEFINITION_CONTEXT ( 'detailed design', #17331, 'design' ) ;
#42778=CARTESIAN_POINT ( 'NONE',  ( -69.17557446582597436, -9.021883352441653514, 7.567125991932351248 ) ) ;
#42794=CARTESIAN_POINT ( 'NONE',  ( -68.87050791938486327, -8.585715889274700530, -6.450409451741323075 ) ) ;
#42821=CARTESIAN_POINT ( 'NONE',  ( 5.057731014323089802, -1.114607557371862567, -2.289010529401726224 ) ) ;
#42830=B_SPLINE_CURVE_WITH_KNOTS ( 'NONE', 3,
 ( #53255, #27111, #44416, #22302, #709, #5813, #1554 ),
 .UNSPECIFIED., .F., .F.,
 ( 4, 3, 4 ),
 ( 0.000000000000000000, 0.0007529153636991639358, 0.001137651663043191038 ),
 .UNSPECIFIED. ) ;
#42850=CARTESIAN_POINT ( 'NONE',  ( -65.60662997296927301, -1.821459649775648396E-14, 0.6641167203969936539 ) ) ;
#42859=VECTOR ( 'NONE', #47738, 1000.000000000000114 ) ;
#42881=FILL_AREA_STYLE ('',( #43710 ) ) ;
#42947=CARTESIAN_POINT ( 'NONE',  ( -68.47885788718261324, 1.837926688830805233, 7.469119143268239114 ) ) ;
#42953=VERTEX_POINT ( 'NONE', #43189 ) ;
#42964=DIRECTION ( 'NONE',  ( -0.000000000000000000, -1.000000000000000000, -0.000000000000000000 ) ) ;
#42969=CARTESIAN_POINT ( 'NONE',  ( -67.27285806668032819, 2.000000000017658319, 1.402349447196803434 ) ) ;
#42974=CARTESIAN_POINT ( 'NONE',  ( -67.03575697379285714, -0.6010133368208401272, -0.6652792357935631840 ) ) ;
#43032=CARTESIAN_POINT ( 'NONE',  ( 5.454592090961234874, -6.230699628392517120, -2.061810099490657411 ) ) ;
#43145=EDGE_LOOP ( 'NONE', ( #42228, #48335, #46403, #4404 ) ) ;
#43189=CARTESIAN_POINT ( 'NONE',  ( 4.866417447938705898, 0.000000000000000000, -1.967953638240998337 ) ) ;
#43208=VERTEX_POINT ( 'NONE', #11026 ) ;
#43222=ORIENTED_EDGE ( 'NONE', *, *, #32733, .T. ) ;
#43280=CARTESIAN_POINT ( 'NONE',  ( -65.41140007701454806, 2.000000000000004441, 1.620203490765837362 ) ) ;
#43385=CARTESIAN_POINT ( 'NONE',  ( 5.617911074533876281, -1.049994927612889040, -2.260412882205727669 ) ) ;
#43387=CARTESIAN_POINT ( 'NONE',  ( -69.34563465300942653, -11.65986150400551580, 7.856885134693455619 ) ) ;
#43429=VERTEX_POINT ( 'NONE', #43935 ) ;
#43443=CARTESIAN_POINT ( 'NONE',  ( -69.93390552824286033, -0.8671508776962656428, -7.500305896622813329 ) ) ;
#43486=CARTESIAN_POINT ( 'NONE',  ( -67.27731269685068582, -9.409571107119717226, -7.454891809856700746 ) ) ;
#43503=DIRECTION ( 'NONE',  ( -0.1139275668495183524, 0.9934890585767659488, 4.694855797473114533E-16 ) ) ;
#43551=EDGE_CURVE ( 'NONE', #39622, #13853, #5038, .T. ) ;
#43593=CYLINDRICAL_SURFACE ( 'NONE', #16479, 0.2499999999999998612 ) ;
#43608=VERTEX_POINT ( 'NONE', #50140 ) ;
#43639=CARTESIAN_POINT ( 'NONE',  ( -69.66748085948010782, -11.69676896150251011, 8.217082732571148185 ) ) ;
#43663=CARTESIAN_POINT ( 'NONE',  ( -69.43545830293986398, -9.790829293527439248, 7.501778215771295777 ) ) ;
#43677=VERTEX_POINT ( 'NONE', #3839 ) ;
#43679=CARTESIAN_POINT ( 'NONE',  ( -65.63888213997375942, -3.295974604355933479E-14, -1.301894315629612997 ) ) ;
#43698=ORIENTED_EDGE ( 'NONE', *, *, #55337, .T. ) ;
#43710=FILL_AREA_STYLE_COLOUR ( '', #6284 ) ;
#43862=DIRECTION ( 'NONE',  ( -0.05705673239519651330, 0.9983709377222391712, 2.351258244848514932E-16 ) ) ;
#43935=CARTESIAN_POINT ( 'NONE',  ( 5.282355347525632183, -1.069580340602398705, -2.393146392891059460 ) ) ;
#43953=CARTESIAN_POINT ( 'NONE',  ( -69.32931325251749399, -9.778513531655887547, 7.370754069753730597 ) ) ;
#44101=CARTESIAN_POINT ( 'NONE',  ( -66.29759486836289284, 1.999999999999978462, 5.111569279459581061 ) ) ;
#44132=DIRECTION ( 'NONE',  ( -0.05705673239519651330, 0.9983709377222391712, 2.351258244848514932E-16 ) ) ;
#44133=DIRECTION ( 'NONE',  ( -0.4165485852472818884, -0.02380568209675183733, -0.9088017196442776946 ) ) ;
#44167=CARTESIAN_POINT ( 'NONE',  ( -66.57154759241068120, -8.723685910846755931, -0.6652792357935665146 ) ) ;
#44199=ORIENTED_EDGE ( 'NONE', *, *, #10714, .T. ) ;
#44205=VERTEX_POINT ( 'NONE', #41827 ) ;
#44229=CARTESIAN_POINT ( 'NONE',  ( 5.283701512688073976, -1.082329719221734932, -2.393429442024904485 ) ) ;
#44247=CARTESIAN_POINT ( 'NONE',  ( -69.33845141029836157, 1.348542913706229918, -7.487543234984622487 ) ) ;
#44252=CARTESIAN_POINT ( 'NONE',  ( -67.98277075215574428, -9.624319141569721126, 5.224814904089846834 ) ) ;
#44255=EDGE_CURVE ( 'NONE', #563, #55181, #49398, .T. ) ;
#44270=CARTESIAN_POINT ( 'NONE',  ( -67.31341032591832629, -9.413710574012958077, -5.859509639694563177 ) ) ;
#44323=CYLINDRICAL_SURFACE ( 'NONE', #47727, 0.2499999999999998612 ) ;
#44328=CARTESIAN_POINT ( 'NONE',  ( 0.09621548157177368943, -1.683565401097097958, 2.124999999999999556 ) ) ;
#44353=CARTESIAN_POINT ( 'NONE',  ( -67.08121593252555215, -9.520946988596053373, 2.735910648343088614 ) ) ;
#44381=ORIENTED_EDGE ( 'NONE', *, *, #34447, .F. ) ;
#44394=FACE_OUTER_BOUND ( 'NONE', #55790, .T. ) ;
#44416=CARTESIAN_POINT ( 'NONE',  ( -70.05831411642593309, -0.4999789778861470357, -7.502972407220384277 ) ) ;
#44422=CARTESIAN_POINT ( 'NONE',  ( -69.11683642851026832, -9.015837829197110409, 7.493101075386320531 ) ) ;
#44492=CARTESIAN_POINT ( 'NONE',  ( -70.56555449637278343, -1.000000000000001776, -8.047023921085740383 ) ) ;
#44501=FACE_OUTER_BOUND ( 'NONE', #25208, .T. ) ;
#44539=EDGE_CURVE ( 'NONE', #9189, #18, #16254, .T. ) ;
#44554=DIRECTION ( 'NONE',  ( -0.9934890585767658377, -0.1139275668495182969, 0.000000000000000000 ) ) ;
#44568=EDGE_CURVE ( 'NONE', #42953, #47190, #3276, .T. ) ;
#44615=CARTESIAN_POINT ( 'NONE',  ( -67.38907591727327429, -11.43549468865002972, -4.725549651853786948 ) ) ;
#44622=DIRECTION ( 'NONE',  ( 2.551063935260010306E-17, -5.102127870520020982E-16, 1.000000000000000000 ) ) ;
#44719=VECTOR ( 'NONE', #37696, 999.9999999999998863 ) ;
#44755=CIRCLE ( 'NONE', #32075, 3.000000000000001332 ) ;
#44758=CARTESIAN_POINT ( 'NONE',  ( 5.558065546916891364, 8.867787166497208620E-06, 2.260478567416572826 ) ) ;
#44759=CARTESIAN_POINT ( 'NONE',  ( -68.26837592669477317, -11.12930981495617644, -7.480194822499078633 ) ) ;
#44816=CARTESIAN_POINT ( 'NONE',  ( -67.52981462395439394, -9.438526564586886991, -7.865887534710968687 ) ) ;
#44821=CYLINDRICAL_SURFACE ( 'NONE', #1083, 0.2499999999999998612 ) ;
#44863=FACE_OUTER_BOUND ( 'NONE', #10113, .T. ) ;
#44923=CARTESIAN_POINT ( 'NONE',  ( -66.59666794111869592, -11.34462593484436077, -7.222001337329467141 ) ) ;
#44927=CARTESIAN_POINT ( 'NONE',  ( -68.86577260744199691, -0.6013940400650622520, -6.479403174770926199 ) ) ;
#44930=CARTESIAN_POINT ( 'NONE',  ( 5.454418722303246092, 0.000000000000000000, -2.500028562687453437 ) ) ;
#45010=CARTESIAN_POINT ( 'NONE',  ( -67.44329683095881478, -8.823711483744059336, 4.584835828370195543 ) ) ;
#45023=CARTESIAN_POINT ( 'NONE',  ( 5.558065690504402134, 8.867811663421879681E-06, -2.260478214935544017 ) ) ;
#45088=CARTESIAN_POINT ( 'NONE',  ( -67.50725361308181505, -1.000000000000000444, 2.158836163547857900 ) ) ;
#45094=CARTESIAN_POINT ( 'NONE',  ( -69.63446883681038457, 1.041039752757419556, -7.493887922408439373 ) ) ;
#45096=CARTESIAN_POINT ( 'NONE',  ( 0.3240706152708103804, -3.670543518250629855, 2.124999999999998668 ) ) ;
#45099=CARTESIAN_POINT ( 'NONE',  ( -68.87050791938486327, -8.585715889274698753, -6.450409451741323075 ) ) ;
#45113=VERTEX_POINT ( 'NONE', #18168 ) ;
#45193=VECTOR ( 'NONE', #53634, 1000.000000000000114 ) ;
#45201=CARTESIAN_POINT ( 'NONE',  ( -64.93522747905139170, -11.15410157257325885, 3.192571262229372930 ) ) ;
#45205=CARTESIAN_POINT ( 'NONE',  ( -67.13674736183641301, -0.6010214343564760364, -1.700609907706588375 ) ) ;
#45218=CARTESIAN_POINT ( 'NONE',  ( -65.70692426961275601, 2.000000000000016875, 3.244935472805978272 ) ) ;
#45235=ORIENTED_EDGE ( 'NONE', *, *, #27467, .T. ) ;
#45274=CARTESIAN_POINT ( 'NONE',  ( -69.18604761972393646, -0.9999999999995233813, 6.394134653913046584 ) ) ;
#45287=FACE_OUTER_BOUND ( 'NONE', #26713, .T. ) ;
#45323=FACE_OUTER_BOUND ( 'NONE', #19177, .T. ) ;
#45343=CARTESIAN_POINT ( 'NONE',  ( -69.95828321977570852, 0.4135283891523413025, -7.500828395702385798 ) ) ;
#45351=ORIENTED_EDGE ( 'NONE', *, *, #44539, .T. ) ;
#45407=VERTEX_POINT ( 'NONE', #29792 ) ;
#45453=CARTESIAN_POINT ( 'NONE',  ( -64.59009247688742050, -11.11452349097115366, 0.8132580553616088892 ) ) ;
#45457=CARTESIAN_POINT ( 'NONE',  ( -66.62196108082586932, 2.602085213965210642E-15, -5.205015551671701601 ) ) ;
#45508=( LENGTH_UNIT ( ) NAMED_UNIT ( * ) SI_UNIT ( .MILLI., .METRE. ) );
#45528=CARTESIAN_POINT ( 'NONE',  ( -69.30403031588791407, -1.000000000000000222, -6.450409451741321298 ) ) ;
#45594=AXIS2_PLACEMENT_3D ( 'NONE', #53023, #9289, #23218 ) ;
#45607=CARTESIAN_POINT ( 'NONE',  ( -58.00000000000000711, 0.000000000000000000, 7.102951435054649637E-15 ) ) ;
#45636=EDGE_LOOP ( 'NONE', ( #5088, #20087 ) ) ;
#45641=CARTESIAN_POINT ( 'NONE',  ( -65.90562112943153750, -9.252273468653816835, -0.3573205173235035614 ) ) ;
#45650=EDGE_CURVE ( 'NONE', #32512, #1529, #1668, .T. ) ;
#45730=B_SPLINE_CURVE_WITH_KNOTS ( 'NONE', 3,
 ( #3346, #37985, #55288, #16378, #33703, #51018, #12129, #29466, #46787, #44759, #31715, #35151, #761, #5034, #27430, #4735 ),
 .UNSPECIFIED., .F., .F.,
 ( 4, 2, 2, 2, 2, 2, 2, 4 ),
 ( 1.734723475976805554E-18, 0.0004228030555968900176, 0.0008456061111937783004, 0.001268409166790666637, 0.001691212222387554866, 0.002114015277984443095, 0.002536818333581331540, 0.003382424444775107997 ),
 .UNSPECIFIED. ) ;
#45735=CARTESIAN_POINT ( 'NONE',  ( -68.36714757807160936, -11.54765427770263742, -6.539696485987661845 ) ) ;
#45740=CARTESIAN_POINT ( 'NONE',  ( -68.22318098944886344, -0.6012227279448117967, -5.285932311688715579 ) ) ;
#45758=CARTESIAN_POINT ( 'NONE',  ( -69.66347483736342383, -8.676648739292067702, -7.503912900124009688 ) ) ;
#45831=CARTESIAN_POINT ( 'NONE',  ( -69.18094373452092327, -0.6002176455286792889, -6.959823595413027419 ) ) ;
#45842=CARTESIAN_POINT ( 'NONE',  ( 5.540715933951533501, -1.051609115606587652, -2.373726444132762570 ) ) ;
#45860=ORIENTED_EDGE ( 'NONE', *, *, #4511, .T. ) ;
#45872=ORIENTED_EDGE ( 'NONE', *, *, #34447, .T. ) ;
#45893=CARTESIAN_POINT ( 'NONE',  ( 4.854282358214435433, 0.000000000000000000, -1.997863978257567785 ) ) ;
#45906=CARTESIAN_POINT ( 'NONE',  ( -57.52614991588065152, -8.291364278369167451, 5.150256511358686722E-15 ) ) ;
#45911=EDGE_CURVE ( 'NONE', #55181, #54422, #35499, .T. ) ;
#45932=ADVANCED_FACE ( 'NONE', ( #16942 ), #43593, .T. ) ;
#45944=CARTESIAN_POINT ( 'NONE',  ( -65.92143918783402512, -9.254087391918899286, 0.7134948435226668995 ) ) ;
#46001=ORIENTED_EDGE ( 'NONE', *, *, #14063, .F. ) ;
#46005=CARTESIAN_POINT ( 'NONE',  ( -65.30511315870414535, -9.183410695202670837, -2.610734445418878558 ) ) ;
#46020=CARTESIAN_POINT ( 'NONE',  ( 5.283695459130013816, -1.082272386734702607, -2.393428169181708309 ) ) ;
#46101=EDGE_CURVE ( 'NONE', #7825, #18, #4407, .T. ) ;
#46102=CARTESIAN_POINT ( 'NONE',  ( -68.84530413953069683, 2.000000000000001776, -6.094799798532269719 ) ) ;
#46180=CARTESIAN_POINT ( 'NONE',  ( -66.26160924740132430, -9.293096122682349858, -3.456045872278597830 ) ) ;
#46192=CARTESIAN_POINT ( 'NONE',  ( 5.558065546916891364, 8.867787166497208620E-06, 2.260478567416572826 ) ) ;
#46197=CARTESIAN_POINT ( 'NONE',  ( -68.43013375671482379, -9.541769944318687635, 7.657917462034228073 ) ) ;
#46205=EDGE_CURVE ( 'NONE', #29912, #25311, #52799, .T. ) ;
#46248=EDGE_LOOP ( 'NONE', ( #128, #24726, #2964, #44199 ) ) ;
#46251=CARTESIAN_POINT ( 'NONE',  ( -66.91922558340073124, -9.368507752467420957, 6.901237005686191139 ) ) ;
#46330=DIRECTION ( 'NONE',  ( -0.9932609354084158682, -0.1139014070068027351, 0.02142857142857155367 ) ) ;
#46347=CARTESIAN_POINT ( 'NONE',  ( -67.39308507045382157, 0.1330233015420136389, 1.352000712394435311 ) ) ;
#46359=CARTESIAN_POINT ( 'NONE',  ( -68.93342745996714882, -0.9999999999999978906, -5.847034362371242189 ) ) ;
#46370=CARTESIAN_POINT ( 'NONE',  ( -67.30190987268471758, -0.6009080523669287910, 2.678990660366964871 ) ) ;
#46391=B_SPLINE_CURVE_WITH_KNOTS ( 'NONE', 3,
 ( #29836, #42594, #43443, #26134 ),
 .UNSPECIFIED., .F., .F.,
 ( 4, 4 ),
 ( 0.0009679422276756598567, 0.001611251064783924929 ),
 .UNSPECIFIED. ) ;
#46403=ORIENTED_EDGE ( 'NONE', *, *, #29162, .T. ) ;
#46445=CARTESIAN_POINT ( 'NONE',  ( -67.14101802347384762, -8.387388012353506284, -2.442027903730112026 ) ) ;
#46472=CARTESIAN_POINT ( 'NONE',  ( -68.77136691953549530, -8.975737434388888047, 7.030741166004676579 ) ) ;
#46490=EDGE_LOOP ( 'NONE', ( #15518, #28424 ) ) ;
#46493=CIRCLE ( 'NONE', #26570, 2.125000000000000000 ) ;
#46543=CARTESIAN_POINT ( 'NONE',  ( -65.69080466243542560, -1.561251128379126069E-14, 1.648866456817433823 ) ) ;
#46556=ADVANCED_FACE ( 'NONE', ( #51068, #38024, #15879 ), #41702, .F. ) ;
#46584=LINE ( 'NONE', #33282, #6112 ) ;
#46635=FACE_OUTER_BOUND ( 'NONE', #43145, .T. ) ;
#46662=CARTESIAN_POINT ( 'NONE',  ( -67.39221309084119582, 0.1329240779904678482, -1.367029069770140604 ) ) ;
#46706=VERTEX_POINT ( 'NONE', #13580 ) ;
#46756=CARTESIAN_POINT ( 'NONE',  ( -66.90530812237336988, -8.360358167099661841, 0.5932824550257441709 ) ) ;
#46784=CARTESIAN_POINT ( 'NONE',  ( -66.02452298553313881, -9.265908444350362316, -1.783245832582586177 ) ) ;
#46787=CARTESIAN_POINT ( 'NONE',  ( -68.51814297103354079, -10.99829263872246088, -7.485193420789068242 ) ) ;
#46836=ORIENTED_EDGE ( 'NONE', *, *, #19840, .T. ) ;
#46962=CARTESIAN_POINT ( 'NONE',  ( -65.88684560494814946, 1.999999999999989120, -3.942473205312013285 ) ) ;
#46964=EDGE_LOOP ( 'NONE', ( #39204, #24973 ) ) ;
#46965=CARTESIAN_POINT ( 'NONE',  ( -69.59775774058348929, -0.6007421665236040154, 7.493101075386322307 ) ) ;
#47026=EDGE_LOOP ( 'NONE', ( #47976, #18547, #15847, #3057 ) ) ;
#47038=CARTESIAN_POINT ( 'NONE',  ( -67.08542992444135677, -8.381013491352103273, 2.158836163547856124 ) ) ;
#47057=CARTESIAN_POINT ( 'NONE',  ( 5.523400220244046643, 0.000000000000000000, 2.340280168031445562 ) ) ;
#47107=( BOUNDED_SURFACE ( )  B_SPLINE_SURFACE ( 3, 2, ( 
 ( #22376, #35162, #9284 ),
 ( #44229, #13556, #43385 ),
 ( #30868, #26605, #31148 ),
 ( #48469, #9592, #1031 ) ),
 .UNSPECIFIED., .F., .F., .F. ) 
 B_SPLINE_SURFACE_WITH_KNOTS ( ( 4, 4 ),
 ( 3, 3 ),
 ( 0.5110550755831337888, 0.5110755313919185250 ),
 ( 0.000000000000000000, 1.000000000000000000 ),
 .UNSPECIFIED. ) 
 GEOMETRIC_REPRESENTATION_ITEM ( )  RATIONAL_B_SPLINE_SURFACE ( (
 ( 1.000000000000000000, 0.6915731974592014275, 1.000000000000000000),
 ( 1.000000000000000000, 0.6915635181374664153, 1.000000000000000000),
 ( 1.000000000000000000, 0.6915538386379234126, 1.000000000000000000),
 ( 1.000000000000000000, 0.6915441589605814121, 1.000000000000000000) ) ) 
 REPRESENTATION_ITEM ( '' )  SURFACE ( )  );
#47111=LINE ( 'NONE', #51651, #22166 ) ;
#47187=CIRCLE ( 'NONE', #16375, 2.125000000000000000 ) ;
#47190=VERTEX_POINT ( 'NONE', #48137 ) ;
#47212=DIRECTION ( 'NONE',  ( -0.1139275668495183524, 0.9934890585767659488, 4.694855797473114533E-16 ) ) ;
#47216=CARTESIAN_POINT ( 'NONE',  ( -67.39666695391619555, 0.1330242493074720589, 1.387855868234969092 ) ) ;
#47234=CARTESIAN_POINT ( 'NONE',  ( 0.000000000000000000, 0.000000000000000000, 0.000000000000000000 ) ) ;
#47260=ORIENTED_EDGE ( 'NONE', *, *, #43551, .T. ) ;
#47265=UNCERTAINTY_MEASURE_WITH_UNIT (LENGTH_MEASURE( 1.000000000000000082E-05 ), #45508, 'distance_accuracy_value', 'NONE');
#47282=ORIENTED_EDGE ( 'NONE', *, *, #19870, .T. ) ;
#47301=ORIENTED_EDGE ( 'NONE', *, *, #21864, .T. ) ;
#47329=EDGE_CURVE ( 'NONE', #563, #27821, #32636, .T. ) ;
#47342=CARTESIAN_POINT ( 'NONE',  ( -69.29498278149517887, -11.65405304096510086, -7.815307374640577898 ) ) ;
#47380=EDGE_LOOP ( 'NONE', ( #39747, #50919, #36998, #47690 ) ) ;
#47383=DIRECTION ( 'NONE',  ( -0.9031405107545327215, -0.1035669190568590248, -0.4166666666666675178 ) ) ;
#47429=FACE_OUTER_BOUND ( 'NONE', #54847, .T. ) ;
#47458=AXIS2_PLACEMENT_3D ( 'NONE', #17455, #29410, #22000 ) ;
#47508=CARTESIAN_POINT ( 'NONE',  ( -68.55686626046413323, 0.1328883920391356610, -5.294842188084643908 ) ) ;
#47519=EDGE_CURVE ( 'NONE', #43608, #11345, #51647, .T. ) ;
#47579=CARTESIAN_POINT ( 'NONE',  ( -1.246832498358330099E-15, 2.000000000000000000, 0.000000000000000000 ) ) ;
#47581=AXIS2_PLACEMENT_3D ( 'NONE', #3361, #20679, #37994 ) ;
#47690=ORIENTED_EDGE ( 'NONE', *, *, #9239, .F. ) ;
#47692=CARTESIAN_POINT ( 'NONE',  ( -65.82994354660264946, -3.295974604355934110E-14, -2.610734445418879002 ) ) ;
#47727=AXIS2_PLACEMENT_3D ( 'NONE', #18184, #35260, #22181 ) ;
#47738=DIRECTION ( 'NONE',  ( 0.05705673239519651330, -0.9983709377222390602, -2.388043913193231768E-16 ) ) ;
#47769=ORIENTED_EDGE ( 'NONE', *, *, #38437, .F. ) ;
#47946=CARTESIAN_POINT ( 'NONE',  ( -67.23718175846519784, -9.538746327908999234, 3.332842667189706898 ) ) ;
#47961=CARTESIAN_POINT ( 'NONE',  ( -67.81506811452879901, 0.000000000000000000, -7.454891809856698970 ) ) ;
#47965=ORIENTED_EDGE ( 'NONE', *, *, #13925, .F. ) ;
#47976=ORIENTED_EDGE ( 'NONE', *, *, #8809, .F. ) ;
#47980=( GEOMETRIC_REPRESENTATION_CONTEXT ( 3 ) GLOBAL_UNCERTAINTY_ASSIGNED_CONTEXT ( ( #54139 ) ) GLOBAL_UNIT_ASSIGNED_CONTEXT ( ( #15629, #50281, #11394 ) ) REPRESENTATION_CONTEXT ( 'NONE', 'WORKASPACE' ) );
#47990=SHAPE_REPRESENTATION_RELATIONSHIP ( 'NONE' , 'NONE' ,  #53575, #3559 ) ;
#48029=DIRECTION ( 'NONE',  ( -0.1139275668495183524, 0.9934890585767659488, 4.694855797473114533E-16 ) ) ;
#48098=( BOUNDED_CURVE ( )  B_SPLINE_CURVE ( 3, ( #5225, #10022, #35576, #27071 ),
 .UNSPECIFIED., .F., .F. ) 
 B_SPLINE_CURVE_WITH_KNOTS ( ( 4, 4 ),
 ( -8.881784197001252323E-16, 1.140403016137402359 ),
 .UNSPECIFIED. ) 
 CURVE ( )  GEOMETRIC_REPRESENTATION_ITEM ( )  RATIONAL_B_SPLINE_CURVE ( ( 1.000000000000000000, 0.8945281452387661147, 0.8945281452387661147, 1.000000000000000000 ) ) 
 REPRESENTATION_ITEM ( '' )  );
#48116=FACE_OUTER_BOUND ( 'NONE', #3295, .T. ) ;
#48130=DIRECTION ( 'NONE',  ( -0.1139275668495183524, 0.9934890585767659488, 4.694855797473114533E-16 ) ) ;
#48137=CARTESIAN_POINT ( 'NONE',  ( 4.930947970565946470, -1.129146301979396139, -1.967953638240999670 ) ) ;
#48147=ORIENTED_EDGE ( 'NONE', *, *, #4151, .T. ) ;
#48258=EDGE_CURVE ( 'NONE', #32717, #13662, #31428, .T. ) ;
#48284=VERTEX_POINT ( 'NONE', #25521 ) ;
#48306=ORIENTED_EDGE ( 'NONE', *, *, #10714, .F. ) ;
#48335=ORIENTED_EDGE ( 'NONE', *, *, #26638, .T. ) ;
#48370=FACE_OUTER_BOUND ( 'NONE', #31505, .T. ) ;
#48416=CARTESIAN_POINT ( 'NONE',  ( 5.454439161952889137, 0.000000000000000000, 2.500037857468615510 ) ) ;
#48469=CARTESIAN_POINT ( 'NONE',  ( 5.282343268243065104, -1.069465939554116174, -2.393143853048730119 ) ) ;
#48475=VECTOR ( 'NONE', #3625, 1000.000000000000114 ) ;
#48486=FACE_OUTER_BOUND ( 'NONE', #47380, .T. ) ;
#48494=DIRECTION ( 'NONE',  ( 0.000000000000000000, 0.000000000000000000, -1.000000000000000000 ) ) ;
#48522=CARTESIAN_POINT ( 'NONE',  ( -69.17625094509207884, -9.022378817169743215, -7.568661514997564232 ) ) ;
#48543=CIRCLE ( 'NONE', #1352, 3.000000000000001332 ) ;
#48574=CARTESIAN_POINT ( 'NONE',  ( -58.00000000000000711, 2.000000000000000000, 3.000000000000008438 ) ) ;
#48672=CARTESIAN_POINT ( 'NONE',  ( -67.14101802347384762, -8.387388012353506284, -2.442027903730112026 ) ) ;
#48673=B_SPLINE_SURFACE_WITH_KNOTS ( 'NONE', 1, 3, ( 
 ( #41388, #27779, #50158, #45099, #25195, #55839, #46445, #46756, #47038, #2722, #8138, #21184, #42496, #42213 ),
 ( #38509, #3323, #37374, #3586, #33681, #55540, #46180, #16949, #38219, #20895, #28882, #7563, #29740, #16643 ) ),
 .UNSPECIFIED., .F., .F., .F.,
 ( 2, 2 ),
 ( 4, 2, 2, 2, 2, 2, 4 ),
 ( 0.000000000000000000, 1.000000000000000000 ),
 ( 0.000000000000000000, 0.1159099261691615840, 0.2318198523383231680, 0.4636397046766463359, 0.6954595570149695316, 0.9272794093532926718, 1.000000000000000000 ),
 .UNSPECIFIED. ) ;
#48788=CARTESIAN_POINT ( 'NONE',  ( -69.91114979398979301, 1.920123671898648382E-16, -8.803577518029833016 ) ) ;
#48797=CARTESIAN_POINT ( 'NONE',  ( -68.46484361067732038, -9.679563055349168721, 6.116987600435763284 ) ) ;
#48813=DIRECTION ( 'NONE',  ( 2.551063935260010306E-17, -4.081702296416016490E-16, 1.000000000000000000 ) ) ;
#48815=CARTESIAN_POINT ( 'NONE',  ( 5.681647518099907757, -6.217723448642448858, 2.166220689508503661 ) ) ;
#48865=ORIENTED_EDGE ( 'NONE', *, *, #40217, .F. ) ;
#48899=CARTESIAN_POINT ( 'NONE',  ( -67.25083081275441543, -9.540336332378162254, -3.375551560942574358 ) ) ;
#48921=ORIENTED_EDGE ( 'NONE', *, *, #37264, .F. ) ;
#48941=CARTESIAN_POINT ( 'NONE',  ( -68.50231803695028532, -8.543494007632164156, -5.847034362371243965 ) ) ;
#48956=SURFACE_STYLE_USAGE ( .BOTH. , #18871 ) ;
#48970=CARTESIAN_POINT ( 'NONE',  ( -69.11692417668358246, -9.015782624321049710, -7.493102809087829108 ) ) ;
#49025=CARTESIAN_POINT ( 'NONE',  ( -67.79584355022304010, 0.1329320821914128370, -3.347029521210270531 ) ) ;
#49027=DIRECTION ( 'NONE',  ( -0.05705673239519650636, 0.9983709377222390602, 2.351258244848514932E-16 ) ) ;
#49038=CARTESIAN_POINT ( 'NONE',  ( -69.75862673655984736, 5.509042946743876566E-16, 8.593930712158172724 ) ) ;
#49071=CARTESIAN_POINT ( 'NONE',  ( -65.95191306736235504, -9.257581959793618864, -4.848827299324492301 ) ) ;
#49072=DIRECTION ( 'NONE',  ( -0.9983709377222390602, -0.05705673239519638146, 0.000000000000000000 ) ) ;
#49160=CARTESIAN_POINT ( 'NONE',  ( -66.00830372752703568, -11.27715573706296404, -6.184885810267199524 ) ) ;
#49165=CARTESIAN_POINT ( 'NONE',  ( -67.13867486860780787, -0.6008876313341391384, 1.704803601115378431 ) ) ;
#49180=CARTESIAN_POINT ( 'NONE',  ( -65.33751984935661028, 2.000000000000018652, -1.324960789524834315 ) ) ;
#49244=CARTESIAN_POINT ( 'NONE',  ( -66.83458874347479650, -8.753654600338279579, -2.670129092015951944 ) ) ;
#49262=CARTESIAN_POINT ( 'NONE',  ( 5.618093201498282063, -1.050357395465043364, -2.260480044901387764 ) ) ;
#49291=EDGE_CURVE ( 'NONE', #50240, #3658, #35178, .T. ) ;
#49295=CIRCLE ( 'NONE', #18480, 6.000000000000001776 ) ;
#49340=FACE_OUTER_BOUND ( 'NONE', #2541, .T. ) ;
#49357=CARTESIAN_POINT ( 'NONE',  ( -67.99506003422921196, -9.491878211616041838, -8.456585623303142896 ) ) ;
#49393=ORIENTED_EDGE ( 'NONE', *, *, #42215, .T. ) ;
#49398=LINE ( 'NONE', #5671, #6806 ) ;
#49444=ADVANCED_FACE ( 'NONE', ( #45287, #27396, #14621 ), #1574, .T. ) ;
#49465=CARTESIAN_POINT ( 'NONE',  ( -65.13797212185212970, -11.17735115307608496, 3.962576710796439805 ) ) ;
#49470=CARTESIAN_POINT ( 'NONE',  ( -66.10170264776731130, 5.898059818321144121E-14, 3.765673540401780262 ) ) ;
#49740=CARTESIAN_POINT ( 'NONE',  ( -66.61623392118266906, 1.734723475976807094E-15, 5.190771789781507550 ) ) ;
#49749=ORIENTED_EDGE ( 'NONE', *, *, #31022, .T. ) ;
#49753=LINE ( 'NONE', #14832, #10534 ) ;
#49796=CARTESIAN_POINT ( 'NONE',  ( -68.83743834501466097, -9.171101568560214190, 7.487530722355575818 ) ) ;
#49807=CARTESIAN_POINT ( 'NONE',  ( -69.23012684808540484, 1.999999999999999112, -6.702751532743288720 ) ) ;
#49818=EDGE_CURVE ( 'NONE', #11345, #10380, #1923, .T. ) ;
#49864=LINE ( 'NONE', #10962, #19280 ) ;
#49889=ORIENTED_EDGE ( 'NONE', *, *, #36334, .F. ) ;
#49898=CARTESIAN_POINT ( 'NONE',  ( -65.19693841791328737, -9.171005842923255713, -1.901374313760128665 ) ) ;
#49923=DIRECTION ( 'NONE',  ( 0.000000000000000000, 0.000000000000000000, 1.000000000000000000 ) ) ;
#49985=CARTESIAN_POINT ( 'NONE',  ( -66.03455808990733544, -11.28016643516713202, 6.196202711025575738 ) ) ;
#49989=CARTESIAN_POINT ( 'NONE',  ( -66.93407535620586657, 2.602085213965210642E-15, -5.905017180572246005 ) ) ;
#50004=LINE ( 'NONE', #38078, #40444 ) ;
#50112=CARTESIAN_POINT ( 'NONE',  ( 5.223256457478859360, -6.243920421220471972, -1.967953638240999670 ) ) ;
#50140=CARTESIAN_POINT ( 'NONE',  ( -69.11692417668358246, -9.015782624321049710, -7.493102809087829108 ) ) ;
#50158=CARTESIAN_POINT ( 'NONE',  ( -69.67957132394272435, -8.678494591075715192, -7.555920072494596518 ) ) ;
#50175=ORIENTED_EDGE ( 'NONE', *, *, #22529, .T. ) ;
#50179=CARTESIAN_POINT ( 'NONE',  ( -66.57362299655956406, -8.724013652710414846, 0.6802539881128697452 ) ) ;
#50211=DIRECTION ( 'NONE',  ( 0.000000000000000000, 1.000000000000000000, 0.000000000000000000 ) ) ;
#50240=VERTEX_POINT ( 'NONE', #36096 ) ;
#50243=CARTESIAN_POINT ( 'NONE',  ( -66.59956646452421580, -9.331851097499329839, -6.325180979151075356 ) ) ;
#50256=CARTESIAN_POINT ( 'NONE',  ( 5.421104749901517472, -1.072937963535797179, 2.456654125669141209 ) ) ;
#50262=EDGE_CURVE ( 'NONE', #51823, #11765, #21328, .T. ) ;
#50281=( NAMED_UNIT ( * ) PLANE_ANGLE_UNIT ( ) SI_UNIT ( $, .RADIAN. ) );
#50283=CARTESIAN_POINT ( 'NONE',  ( -67.69264396058785849, 5.362719954027564582E-12, -5.540714948658928662 ) ) ;
#50329=ORIENTED_EDGE ( 'NONE', *, *, #32481, .T. ) ;
#50393=CARTESIAN_POINT ( 'NONE',  ( -69.24055593166185929, -10.33124374485395514, 7.498947595741733529 ) ) ;
#50486=CARTESIAN_POINT ( 'NONE',  ( -67.12594105347433526, -9.392212684426485936, 7.224227263220592832 ) ) ;
#50584=PLANE ( 'NONE',  #18172 ) ;
#50633=FACE_BOUND ( 'NONE', #46964, .T. ) ;
#50635=CARTESIAN_POINT ( 'NONE',  ( -68.54116703456952564, -9.287124719764433323, 7.481505251583916660 ) ) ;
#50745=CARTESIAN_POINT ( 'NONE',  ( -67.74416038478570101, -8.858064234063045106, 5.268187007955521750 ) ) ;
#50786=LINE ( 'NONE', #32911, #37573 ) ;
#50801=CARTESIAN_POINT ( 'NONE',  ( -65.07102203629978021, -9.156566482107063365, 0.3363546178749044491 ) ) ;
#50833=CARTESIAN_POINT ( 'NONE',  ( -67.62965612898899792, -11.46308303289930386, -8.694190345973900946 ) ) ;
#50893=CARTESIAN_POINT ( 'NONE',  ( -67.33410474092524112, 0.1329883344697675163, 0.6700356180039969134 ) ) ;
#50910=CARTESIAN_POINT ( 'NONE',  ( -68.15691219544618207, 2.000000000026043612, -4.725549651835818210 ) ) ;
#50913=CARTESIAN_POINT ( 'NONE',  ( -68.81473095537231188, -0.6015118236491385773, -6.396357082918164849 ) ) ;
#50919=ORIENTED_EDGE ( 'NONE', *, *, #29746, .T. ) ;
#50926=CARTESIAN_POINT ( 'NONE',  ( -68.13401945688795536, -11.18625196726625148, 7.477472888882759960 ) ) ;
#50940=ORIENTED_EDGE ( 'NONE', *, *, #11548, .T. ) ;
#50966=CARTESIAN_POINT ( 'NONE',  ( 5.558065690504402134, 8.867811663421879681E-06, -2.260478214935544017 ) ) ;
#51016=CARTESIAN_POINT ( 'NONE',  ( -66.20424668929096867, -9.286518117000532868, 2.845885083223566703 ) ) ;
#51018=CARTESIAN_POINT ( 'NONE',  ( -68.96626428157883026, -10.65111260844145313, -7.493887922408438484 ) ) ;
#51068=FACE_OUTER_BOUND ( 'NONE', #51131, .T. ) ;
#51118=CARTESIAN_POINT ( 'NONE',  ( -68.76211497692452213, -11.59294684971063916, -7.108028418031229201 ) ) ;
#51120=ORIENTED_EDGE ( 'NONE', *, *, #22715, .T. ) ;
#51131=EDGE_LOOP ( 'NONE', ( #55302, #36486, #34355, #51795 ) ) ;
#51133=LINE ( 'NONE', #11410, #15017 ) ;
#51154=ADVANCED_FACE ( 'NONE', ( #26715 ), #44323, .T. ) ;
#51189=FACE_OUTER_BOUND ( 'NONE', #30852, .T. ) ;
#51208=CARTESIAN_POINT ( 'NONE',  ( -69.53119166430043663, 1.999999999951586060, 7.127210919673932388 ) ) ;
#51213=CARTESIAN_POINT ( 'NONE',  ( -67.46601601628378830, -0.6012495896919525240, -3.320464512871842189 ) ) ;
#51288=VECTOR ( 'NONE', #56034, 1000.000000000000227 ) ;
#51295=CARTESIAN_POINT ( 'NONE',  ( -57.29829478218162109, -10.27834239552269935, 3.000000000000005773 ) ) ;
#51316=CARTESIAN_POINT ( 'NONE',  ( -57.29829478218162109, -10.27834239552269580, -2.999999999999996891 ) ) ;
#51325=CARTESIAN_POINT ( 'NONE',  ( -66.08210154591968433, -11.28561844313478524, 6.312544413184012271 ) ) ;
#51427=CARTESIAN_POINT ( 'NONE',  ( -67.46615831890672155, 4.336808689942017736E-15, 6.899827505724789312 ) ) ;
#51454=ORIENTED_EDGE ( 'NONE', *, *, #46205, .T. ) ;
#51491=EDGE_CURVE ( 'NONE', #44205, #10708, #24759, .T. ) ;
#51507=CARTESIAN_POINT ( 'NONE',  ( -68.57948186459397277, 0.1329774074821103713, 5.304050906517310260 ) ) ;
#51510=CARTESIAN_POINT ( 'NONE',  ( -69.39314964050831236, -0.6010558250688294857, 7.224037831218162786 ) ) ;
#51513=CARTESIAN_POINT ( 'NONE',  ( 5.284365508485809215, -1.088618427183434934, -2.393569053917001810 ) ) ;
#51600=CARTESIAN_POINT ( 'NONE',  ( 5.454439161952889137, 0.000000000000000000, 2.500037857468615510 ) ) ;
#51625=DIRECTION ( 'NONE',  ( 0.000000000000000000, 1.000000000000000000, -0.000000000000000000 ) ) ;
#51647=B_SPLINE_CURVE_WITH_KNOTS ( 'NONE', 3,
 ( #30513, #9181, #29931, #13461 ),
 .UNSPECIFIED., .F., .F.,
 ( 4, 4 ),
 ( 0.0009679422276756773124, 0.001611251064783924929 ),
 .UNSPECIFIED. ) ;
#51651=CARTESIAN_POINT ( 'NONE',  ( 2.602374448188125350E-16, 2.000000000000000000, 2.125000000000000000 ) ) ;
#51664=CARTESIAN_POINT ( 'NONE',  ( 5.558065690504402134, 8.867811663421879681E-06, -2.260478214935544017 ) ) ;
#51758=CARTESIAN_POINT ( 'NONE',  ( -67.62757635072813400, 0.1329464987405940268, -2.709928232736921405 ) ) ;
#51771=CIRCLE ( 'NONE', #27289, 3.000000000000001332 ) ;
#51795=ORIENTED_EDGE ( 'NONE', *, *, #4274, .F. ) ;
#51823=VERTEX_POINT ( 'NONE', #51316 ) ;
#51864=CARTESIAN_POINT ( 'NONE',  ( 5.446213544912834159, -1.070058632457644654, 0.6896135826588392082 ) ) ;
#51880=CARTESIAN_POINT ( 'NONE',  ( -69.94833770632727976, -8.709315162003530730, 7.852029984319920608 ) ) ;
#51904=CARTESIAN_POINT ( 'NONE',  ( -68.92522653842155478, -9.732315607823066372, 6.824617610603313622 ) ) ;
#51958=SURFACE_STYLE_USAGE ( .BOTH. , #29845 ) ;
#52041=CARTESIAN_POINT ( 'NONE',  ( -68.28917301125578376, 0.1329764677542568940, 4.678579668399310165 ) ) ;
#52120=CARTESIAN_POINT ( 'NONE',  ( -58.00000000000000711, 0.000000000000000000, 3.000000000000008438 ) ) ;
#52263=CARTESIAN_POINT ( 'NONE',  ( 5.618093942130458096, -1.050357310661657939, 2.260478214906367800 ) ) ;
#52322=ORIENTED_EDGE ( 'NONE', *, *, #18047, .F. ) ;
#52380=EDGE_CURVE ( 'NONE', #7825, #48284, #39501, .T. ) ;
#52642=ORIENTED_EDGE ( 'NONE', *, *, #25020, .T. ) ;
#52655=CARTESIAN_POINT ( 'NONE',  ( -66.99903215919390220, -8.772469562030201118, -3.320464512871846186 ) ) ;
#52671=CARTESIAN_POINT ( 'NONE',  ( 5.551076178010876383, -1.058033593491026769, -2.420903799066405071 ) ) ;
#52740=AXIS2_PLACEMENT_3D ( 'NONE', #48815, #13342, #49072 ) ;
#52750=ORIENTED_EDGE ( 'NONE', *, *, #89, .T. ) ;
#52757=EDGE_CURVE ( 'NONE', #47190, #16329, #14776, .T. ) ;
#52773=EDGE_CURVE ( 'NONE', #10380, #16523, #45730, .T. ) ;
#52794=AXIS2_PLACEMENT_3D ( 'NONE', #41143, #18442, #44554 ) ;
#52799=CIRCLE ( 'NONE', #18307, 6.000000000000002665 ) ;
#52810=CARTESIAN_POINT ( 'NONE',  ( 0.1285714285714296967, 2.000000000000000000, 5.998622290806041590 ) ) ;
#52835=DIRECTION ( 'NONE',  ( -2.551063935260010306E-17, 4.081702296416016490E-16, -1.000000000000000000 ) ) ;
#52883=CARTESIAN_POINT ( 'NONE',  ( -67.50810339439870233, 2.000000000000000000, 7.448312483692316022 ) ) ;
#52889=CIRCLE ( 'NONE', #47458, 2.125000000000000000 ) ;
#52911=CARTESIAN_POINT ( 'NONE',  ( -68.01236371044051054, -8.487308885305189676, 5.059064008999122564 ) ) ;
#52932=AXIS2_PLACEMENT_3D ( 'NONE', #31905, #19114, #27359 ) ;
#53023=CARTESIAN_POINT ( 'NONE',  ( 0.000000000000000000, 2.000000000000000000, 0.000000000000000000 ) ) ;
#53174=CARTESIAN_POINT ( 'NONE',  ( -66.50642983938375608, -11.33427795235789226, -1.381457631280774700 ) ) ;
#53191=ORIENTED_EDGE ( 'NONE', *, *, #52757, .F. ) ;
#53196=CARTESIAN_POINT ( 'NONE',  ( -67.15282819338808906, 1.999999999999999556, -6.891906871564128068 ) ) ;
#53223=EDGE_CURVE ( 'NONE', #11765, #51823, #30545, .T. ) ;
#53255=CARTESIAN_POINT ( 'NONE',  ( -70.10219403106212610, -1.000000000000000666, -7.503912900124007912 ) ) ;
#53260=CARTESIAN_POINT ( 'NONE',  ( -66.55938532089209048, -8.722345891443490373, 0.3404743498653450273 ) ) ;
#53316=CARTESIAN_POINT ( 'NONE',  ( -67.62405810989892530, 0.1329463135932536511, -2.692672496485626787 ) ) ;
#53329=CARTESIAN_POINT ( 'NONE',  ( -68.50955275228491814, 4.575831628609406792E-15, -7.038790429923466263 ) ) ;
#53338=CARTESIAN_POINT ( 'NONE',  ( -58.00000000000000711, 2.000000000000000000, 7.102951435054649637E-15 ) ) ;
#53360=ORIENTED_EDGE ( 'NONE', *, *, #52380, .F. ) ;
#53407=CARTESIAN_POINT ( 'NONE',  ( -70.10169143752739274, -0.9999999999999995559, 7.503902134509972122 ) ) ;
#53437=CARTESIAN_POINT ( 'NONE',  ( -64.93003644718953637, -11.15350629512717795, -3.167379070703715271 ) ) ;
#53441=CARTESIAN_POINT ( 'NONE',  ( -65.72105987057051379, -5.204170427930421283E-15, -1.901374313756482026 ) ) ;
#53459=VERTEX_POINT ( 'NONE', #14590 ) ;
#53507=CARTESIAN_POINT ( 'NONE',  ( -68.62489455609114941, -8.958878114863663811, 6.810182420670462200 ) ) ;
#53517=CARTESIAN_POINT ( 'NONE',  ( 6.001673238768763241, 0.0004827855012993410204, 0.7726390298733384343 ) ) ;
#53527=CARTESIAN_POINT ( 'NONE',  ( -67.02814355662815160, -11.39410505754381475, 7.454431982338129536 ) ) ;
#53552=CARTESIAN_POINT ( 'NONE',  ( 4.930947970565944694, -1.129146301979397693, 1.967953638241001446 ) ) ;
#53562=CARTESIAN_POINT ( 'NONE',  ( -68.48130668646780350, 0.1328705276719804873, -5.273316683197703192 ) ) ;
#53574=CARTESIAN_POINT ( 'NONE',  ( -67.92731540425158698, 5.350669522624571327E-13, 6.206396125462542379 ) ) ;
#53575=SHAPE_REPRESENTATION ( 'Curved Precision Cutting Blades', ( #2610 ), #47980 ) ;
#53607=CARTESIAN_POINT ( 'NONE',  ( -67.15568563940774993, -9.395623621142684456, -5.540714948658321148 ) ) ;
#53634=DIRECTION ( 'NONE',  ( -0.05705673239519650636, 0.9983709377222390602, 2.351258244848514932E-16 ) ) ;
#53642=CARTESIAN_POINT ( 'NONE',  ( -67.50725361308181505, -1.000000000000000444, 2.158836163547857900 ) ) ;
#53645=CARTESIAN_POINT ( 'NONE',  ( 4.912750499197527709, -1.131233082521084565, -2.029539223447461627 ) ) ;
#53650=PRODUCT_DEFINITION_SHAPE ( 'NONE', 'NONE',  #25667 ) ;
#53651=LINE ( 'NONE', #10528, #4167 ) ;
#53698=CARTESIAN_POINT ( 'NONE',  ( -68.68338454767959433, -9.704603335163470845, 6.496570960383161619 ) ) ;
#53703=CARTESIAN_POINT ( 'NONE',  ( -67.09538265911608335, -0.6008884158751092164, 1.362417606695038641 ) ) ;
#53776=CARTESIAN_POINT ( 'NONE',  ( -67.50725361308181505, -1.000000000000000000, 2.158836163547857900 ) ) ;
#53796=CARTESIAN_POINT ( 'NONE',  ( 5.282355347525632183, -1.069580340602398705, -2.393146392891059460 ) ) ;
#53801=ORIENTED_EDGE ( 'NONE', *, *, #25576, .T. ) ;
#53802=CARTESIAN_POINT ( 'NONE',  ( -67.72739005747112628, -11.31115511663740136, 7.469119143268238226 ) ) ;
#53841=CARTESIAN_POINT ( 'NONE',  ( 5.204999356530673360, -6.244963811491317074, 2.061810099490656079 ) ) ;
#53907=CARTESIAN_POINT ( 'NONE',  ( 4.866417447938704122, 0.000000000000000000, 1.967953638241001002 ) ) ;
#53948=CARTESIAN_POINT ( 'NONE',  ( 5.592545315101208558, -1.053278153209864065, -2.323295808888600433 ) ) ;
#53951=VECTOR ( 'NONE', #42723, 1000.000000000000000 ) ;
#53995=CARTESIAN_POINT ( 'NONE',  ( -64.58775654058000271, -11.11425561933479855, -0.8023217398921337340 ) ) ;
#53999=CARTESIAN_POINT ( 'NONE',  ( -67.93758966355230200, -0.6009655799177398006, 4.644600239861888191 ) ) ;
#54015=EDGE_CURVE ( 'NONE', #2677, #1529, #18664, .T. ) ;
#54017=CARTESIAN_POINT ( 'NONE',  ( -69.48696977452702583, -9.539949144137821690, -7.502262482362485052 ) ) ;
#54022=AXIS2_PLACEMENT_3D ( 'NONE', #54568, #33015, #46330 ) ;
#54055=SURFACE_STYLE_FILL_AREA ( #1540 ) ;
#54065=CARTESIAN_POINT ( 'NONE',  ( 5.618093201498282063, -1.050357395465043364, -2.260480044901387764 ) ) ;
#54091=DIRECTION ( 'NONE',  ( -0.9934890585767658377, -0.1139275668495182969, 0.000000000000000000 ) ) ;
#54134=CARTESIAN_POINT ( 'NONE',  ( 0.4518049228021099872, -3.655895688227116747, -5.998622290806042479 ) ) ;
#54139=UNCERTAINTY_MEASURE_WITH_UNIT (LENGTH_MEASURE( 1.000000000000000082E-05 ), #15629, 'distance_accuracy_value', 'NONE');
#54184=CARTESIAN_POINT ( 'NONE',  ( -67.54131694805309394, -9.439845584445631488, 7.854170068343406363 ) ) ;
#54188=FACE_OUTER_BOUND ( 'NONE', #4217, .T. ) ;
#54270=CARTESIAN_POINT ( 'NONE',  ( -68.17821258402990736, -9.646719645199189230, 5.608481661906881577 ) ) ;
#54273=CARTESIAN_POINT ( 'NONE',  ( -67.02334604683971975, -0.6009592863103402349, 0.3393403235780959037 ) ) ;
#54340=MECHANICAL_DESIGN_GEOMETRIC_PRESENTATION_REPRESENTATION('',(#10817),#25325);
#54341=CARTESIAN_POINT ( 'NONE',  ( -71.02048890987401819, -0.9999999999999995559, 8.554889286408840832 ) ) ;
#54345=CARTESIAN_POINT ( 'NONE',  ( -68.02073773998908734, 2.000000000000048850, 8.237893588744196194 ) ) ;
#54358=ORIENTED_EDGE ( 'NONE', *, *, #34591, .F. ) ;
#54383=ORIENTED_EDGE ( 'NONE', *, *, #21987, .T. ) ;
#54422=VERTEX_POINT ( 'NONE', #39324 ) ;
#54435=CARTESIAN_POINT ( 'NONE',  ( -65.57510285225123425, -9.214371548364283626, 3.765673540395807706 ) ) ;
#54490=CARTESIAN_POINT ( 'NONE',  ( -65.30888085680906840, -9.183842752983270685, 2.627585852360244445 ) ) ;
#54506=CARTESIAN_POINT ( 'NONE',  ( 5.283025405476269754, -1.075926357871029415, -2.393287282172987140 ) ) ;
#54524=CARTESIAN_POINT ( 'NONE',  ( -66.51057813521288153, 4.515102018714843381E-12, 1.428098984229650759 ) ) ;
#54568=CARTESIAN_POINT ( 'NONE',  ( 0.4518049228021103203, -3.655895688227122076, 5.998622290806040702 ) ) ;
#54599=CARTESIAN_POINT ( 'NONE',  ( -68.92435787895500710, 2.000000000000635048, 6.355103916287438537 ) ) ;
#54610=LINE ( 'NONE', #20569, #42391 ) ;
#54718=CARTESIAN_POINT ( 'NONE',  ( -66.08628404271949819, -9.272990844416433731, 5.190771789778323431 ) ) ;
#54755=CARTESIAN_POINT ( 'NONE',  ( -1.246832498358330099E-15, 0.000000000000000000, 0.000000000000000000 ) ) ;
#54783=CARTESIAN_POINT ( 'NONE',  ( -66.59971854373151245, -9.331868537061321689, 6.321089406856088111 ) ) ;
#54790=CARTESIAN_POINT ( 'NONE',  ( -66.57865728943677652, 2.471980953266950110E-14, 5.126821739293251134 ) ) ;
#54824=CARTESIAN_POINT ( 'NONE',  ( -69.65680208973252263, -0.6014278869996851906, 7.567125991932363682 ) ) ;
#54847=EDGE_LOOP ( 'NONE', ( #27424, #37753, #18974, #35765 ) ) ;
#54892=CARTESIAN_POINT ( 'NONE',  ( -67.78991508493417939, 0.1329061886590362507, 3.332842667189709562 ) ) ;
#54920=CARTESIAN_POINT ( 'NONE',  ( -69.19743948421294988, -0.6012349891692201354, 6.949370683160942974 ) ) ;
#54924=CARTESIAN_POINT ( 'NONE',  ( -69.59783862807636012, -0.6008070088998225255, -7.493102809087827332 ) ) ;
#55002=DIRECTION ( 'NONE',  ( -0.1139275668495183386, 0.9934890585767658377, 4.694855797473113547E-16 ) ) ;
#55027=CARTESIAN_POINT ( 'NONE',  ( -64.58934917682360322, -11.11443825362803395, 0.6542134465202145144 ) ) ;
#55031=CARTESIAN_POINT ( 'NONE',  ( -67.30865983991493806, -9.413165815805299985, 5.846634436079878760 ) ) ;
#55044=CYLINDRICAL_SURFACE ( 'NONE', #40181, 5.991923709989089630 ) ;
#55045=CARTESIAN_POINT ( 'NONE',  ( 5.223256457478858472, -6.243920421220472861, 1.967953638240999670 ) ) ;
#55077=CARTESIAN_POINT ( 'NONE',  ( 0.3240706152708093812, -3.670543518250628967, -1.335466778558061241E-15 ) ) ;
#55086=CARTESIAN_POINT ( 'NONE',  ( -67.27849890436391433, -9.409707134521932304, 7.454917401049827141 ) ) ;
#55124=CARTESIAN_POINT ( 'NONE',  ( 0.3240706152708106025, -3.670543518250628967, -1.335466778558061241E-15 ) ) ;
#55172=PLANE ( 'NONE',  #31903 ) ;
#55174=CARTESIAN_POINT ( 'NONE',  ( -69.20357155325814347, 0.1329212998141634239, 6.404540763468512310 ) ) ;
#55180=DIRECTION ( 'NONE',  ( -0.05705673239519650636, 0.9983709377222390602, 2.328063060706355175E-16 ) ) ;
#55181=VERTEX_POINT ( 'NONE', #26684 ) ;
#55189=CARTESIAN_POINT ( 'NONE',  ( -67.80365641637717999, 0.1329308371501277952, -3.375551560958620634 ) ) ;
#55192=CARTESIAN_POINT ( 'NONE',  ( -68.65415923196773917, -0.6013102719389076256, 6.097755213354411730 ) ) ;
#55281=ORIENTED_EDGE ( 'NONE', *, *, #47519, .F. ) ;
#55286=CARTESIAN_POINT ( 'NONE',  ( -65.08541935831070191, -9.158217483546630788, -0.7600040867655236676 ) ) ;
#55288=CARTESIAN_POINT ( 'NONE',  ( -69.35946117089058305, -10.06457831932934965, -7.500828395702386686 ) ) ;
#55302=ORIENTED_EDGE ( 'NONE', *, *, #30027, .F. ) ;
#55331=DIRECTION ( 'NONE',  ( -2.683102249366423030E-17, 4.694855797473116505E-16, -1.000000000000000000 ) ) ;
#55337=EDGE_CURVE ( 'NONE', #17834, #43208, #31790, .T. ) ;
#55343=CARTESIAN_POINT ( 'NONE',  ( -65.44640951980584020, -9.199613742922251092, -3.251835480715623117 ) ) ;
#55351=ORIENTED_EDGE ( 'NONE', *, *, #37182, .F. ) ;
#55457=CARTESIAN_POINT ( 'NONE',  ( -69.84500490485720547, 0.1331119800031512479, -7.306024462449258294 ) ) ;
#55504=EDGE_CURVE ( 'NONE', #43608, #3029, #38662, .T. ) ;
#55514=CARTESIAN_POINT ( 'NONE',  ( 5.454418722303246092, 0.000000000000000000, -2.500028562687453437 ) ) ;
#55540=CARTESIAN_POINT ( 'NONE',  ( -66.80814951898862830, -9.355770193211530028, -5.009371237985869918 ) ) ;
#55554=CARTESIAN_POINT ( 'NONE',  ( -68.90818038468613338, -0.2025580785338727541, 7.478321023991167493 ) ) ;
#55561=CARTESIAN_POINT ( 'NONE',  ( -66.39287224736634130, -11.32125582591041280, 6.891331229949073212 ) ) ;
#55581=CARTESIAN_POINT ( 'NONE',  ( -70.26988861484534254, -8.746188756442855095, 8.208045577613539479 ) ) ;
#55621=CARTESIAN_POINT ( 'NONE',  ( 4.597055792761644888, -1.167435121648761065, 2.076476591771610369 ) ) ;
#55622=CARTESIAN_POINT ( 'NONE',  ( -65.81766060794319628, -9.242186665891644282, -4.508581566067809909 ) ) ;
#55624=AXIS2_PLACEMENT_3D ( 'NONE', #13815, #19480, #27169 ) ;
#55639=ADVANCED_FACE ( 'NONE', ( #23676 ), #40543, .T. ) ;
#55658=ADVANCED_FACE ( 'NONE', ( #4368 ), #37881, .F. ) ;
#55668=CARTESIAN_POINT ( 'NONE',  ( -68.53670954776376334, 2.081668171172168513E-14, 8.455601507725491572 ) ) ;
#55733=ADVANCED_FACE ( 'NONE', ( #29346 ), #25636, .F. ) ;
#55750=CARTESIAN_POINT ( 'NONE',  ( -67.33498797961308924, 0.1329898013568112103, 0.6944083026028426975 ) ) ;
#55755=CARTESIAN_POINT ( 'NONE',  ( -68.82653453192783388, -0.6013598542774325484, 6.387117138744211609 ) ) ;
#55790=EDGE_LOOP ( 'NONE', ( #34621, #39358, #28446, #3597 ) ) ;
#55815=CARTESIAN_POINT ( 'NONE',  ( -58.00000000000000711, 0.000000000000000000, 7.102951435054649637E-15 ) ) ;
#55839=CARTESIAN_POINT ( 'NONE',  ( -67.55782011861325032, -8.435184460786505412, -3.909888324369926060 ) ) ;
#55887=FACE_OUTER_BOUND ( 'NONE', #37077, .T. ) ;
#55900=ORIENTED_EDGE ( 'NONE', *, *, #34203, .F. ) ;
#55930=EDGE_CURVE ( 'NONE', #2677, #16356, #13147, .T. ) ;
#55938=CARTESIAN_POINT ( 'NONE',  ( -65.65478415642573395, -1.821459649775647449E-14, 1.319813854473108838 ) ) ;
#55947=VECTOR ( 'NONE', #492, 1000.000000000000000 ) ;
#55953=DIRECTION ( 'NONE',  ( -0.9983709377222390602, -0.05705673239519638146, 0.000000000000000000 ) ) ;
#56010=ORIENTED_EDGE ( 'NONE', *, *, #10546, .F. ) ;
#56024=ORIENTED_EDGE ( 'NONE', *, *, #16120, .F. ) ;
#56034=DIRECTION ( 'NONE',  ( 0.9090593428863094072, 0.000000000000000000, -0.4166666666666668517 ) ) ;
#56045=CARTESIAN_POINT ( 'NONE',  ( -65.33723405956592956, 1.999999999999986233, -0.8023217398950600598 ) ) ;
#56184=DIRECTION ( 'NONE',  ( -0.9932609354084158682, -0.1139014070068027212, -0.02142857142857160571 ) ) ;
#56198=LINE ( 'NONE', #25531, #24873 ) ;
#56201=CARTESIAN_POINT ( 'NONE',  ( 5.500940387028407486, 0.000000000000000000, -2.400892578144000034 ) ) ;
ENDSEC;
END-ISO-10303-21;
